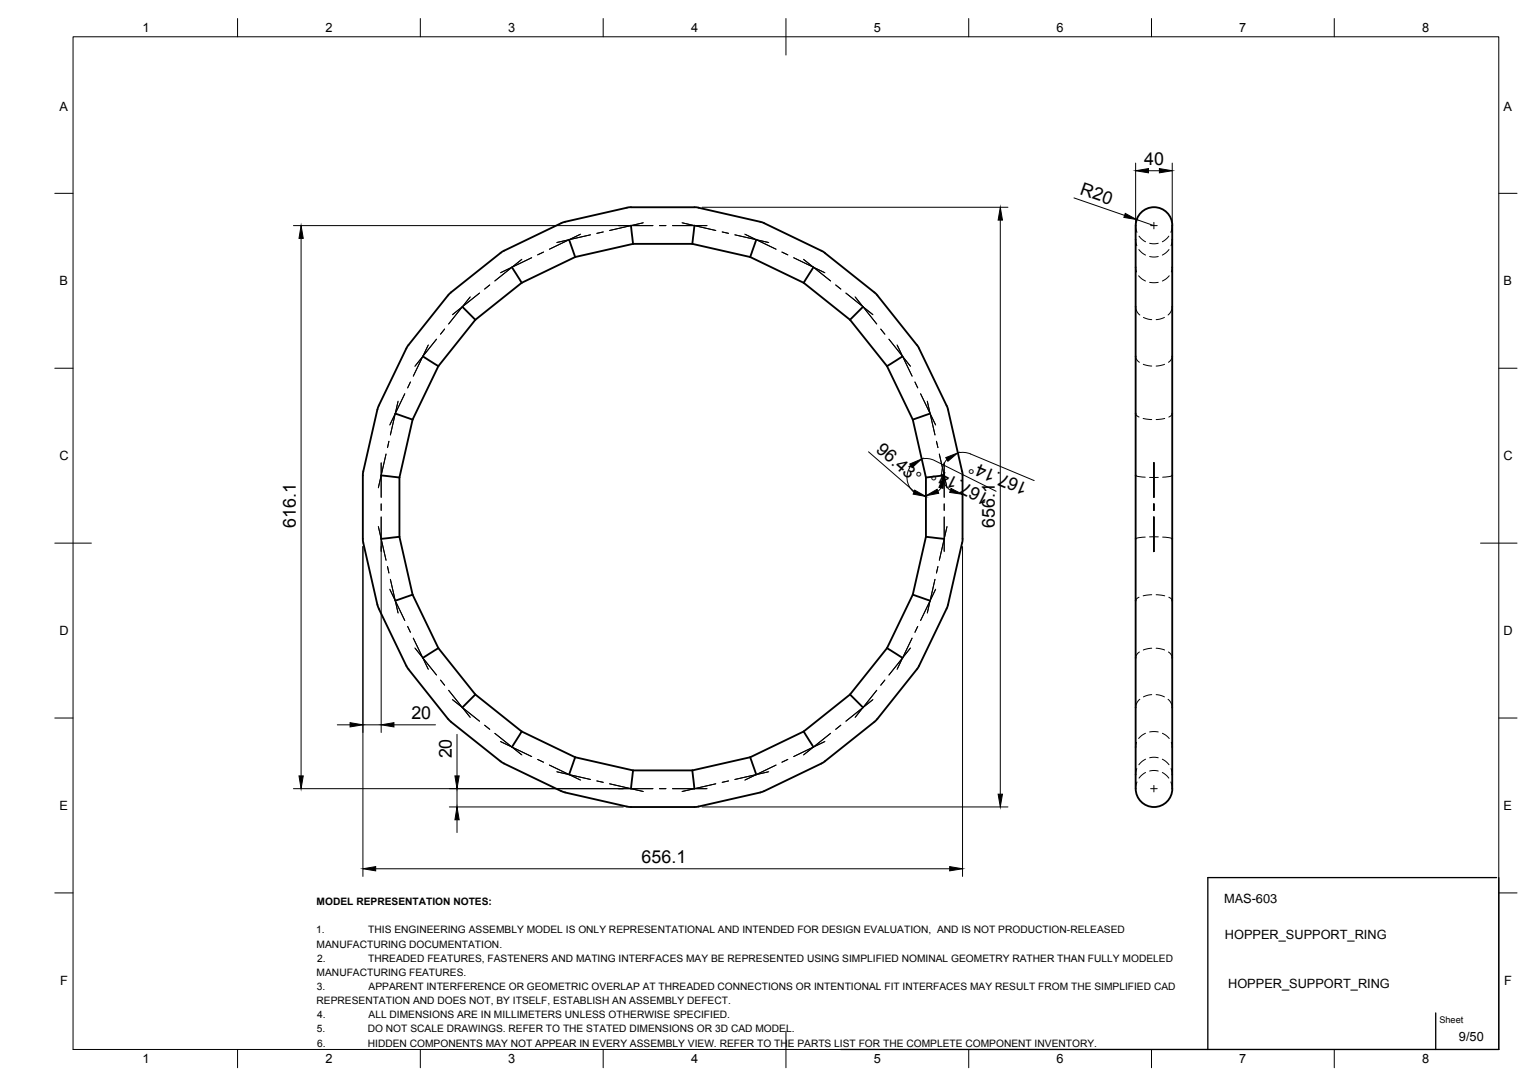
ISO-10303-21;
HEADER;
FILE_DESCRIPTION((''),'2;1');
FILE_NAME('HOPPER_SUPPORT_RING.step','2026-10-01T22:06:14-07:00',(''),(''),'','','');
FILE_SCHEMA (('AUTOMOTIVE_DESIGN { 1 0 10303 214 3 1 1 }'));
ENDSEC;
DATA;
#10=MECHANICAL_DESIGN_GEOMETRIC_PRESENTATION_REPRESENTATION('',(#985),#50440);
#362=ELLIPSE('',#29844,2.01265515316035,2.) ;
#363=ELLIPSE('',#29845,2.01265515316035,2.) ;
#364=ELLIPSE('',#29846,2.01265515316036,2.) ;
#365=ELLIPSE('',#29847,2.01265515316036,2.) ;
#366=ELLIPSE('',#29849,2.01265515316036,2.) ;
#367=ELLIPSE('',#29850,2.01265515316036,2.) ;
#368=ELLIPSE('',#29852,2.01265515316036,2.) ;
#369=ELLIPSE('',#29853,2.01265515316036,2.) ;
#370=ELLIPSE('',#29855,2.01265515316035,2.) ;
#371=ELLIPSE('',#29856,2.01265515316035,2.) ;
#372=ELLIPSE('',#29858,2.01265515316036,2.) ;
#373=ELLIPSE('',#29859,2.01265515316036,2.) ;
#374=ELLIPSE('',#29861,2.01265515316036,2.) ;
#375=ELLIPSE('',#29862,2.01265515316036,2.) ;
#376=ELLIPSE('',#29864,2.01265515316036,2.) ;
#377=ELLIPSE('',#29865,2.01265515316036,2.) ;
#378=ELLIPSE('',#29867,2.01265515316036,2.) ;
#379=ELLIPSE('',#29869,2.01265515316036,2.) ;
#380=ELLIPSE('',#29871,2.01265515316036,2.) ;
#381=ELLIPSE('',#29873,2.01265515316035,2.) ;
#382=ELLIPSE('',#29875,2.01265515316036,2.) ;
#383=ELLIPSE('',#29877,2.01265515316036,2.) ;
#384=ELLIPSE('',#29879,2.01265515316036,2.) ;
#385=ELLIPSE('',#29881,2.01265515316036,2.) ;
#386=ELLIPSE('',#29883,2.01265515316036,2.) ;
#387=ELLIPSE('',#29885,2.01265515316036,2.) ;
#388=ELLIPSE('',#29887,2.01265515316036,2.) ;
#389=ELLIPSE('',#29889,2.01265515316036,2.) ;
#390=ELLIPSE('',#29891,2.01265515316036,2.) ;
#391=ELLIPSE('',#29893,2.01265515316036,2.) ;
#392=ELLIPSE('',#29894,2.01265515316036,2.) ;
#393=ELLIPSE('',#29896,2.01265515316036,2.) ;
#394=ELLIPSE('',#29897,2.01265515316036,2.) ;
#395=ELLIPSE('',#29899,2.01265515316035,2.) ;
#396=ELLIPSE('',#29900,2.01265515316035,2.) ;
#397=ELLIPSE('',#29902,2.01265515316036,2.) ;
#398=ELLIPSE('',#29903,2.01265515316036,2.) ;
#399=ELLIPSE('',#29905,2.01265515316036,2.) ;
#400=ELLIPSE('',#29906,2.01265515316036,2.) ;
#401=ELLIPSE('',#29908,2.01265515316036,2.) ;
#402=ELLIPSE('',#29909,2.01265515316036,2.) ;
#403=ELLIPSE('',#29911,2.01265515316036,2.) ;
#404=ELLIPSE('',#29912,2.01265515316036,2.) ;
#699=SPHERICAL_SURFACE('',#29731,2.) ;
#700=SPHERICAL_SURFACE('',#29734,2.) ;
#701=SPHERICAL_SURFACE('',#29737,2.) ;
#702=SPHERICAL_SURFACE('',#29740,2.) ;
#703=SPHERICAL_SURFACE('',#29743,2.) ;
#704=SPHERICAL_SURFACE('',#29746,2.) ;
#705=SPHERICAL_SURFACE('',#29749,2.) ;
#706=SPHERICAL_SURFACE('',#29752,2.) ;
#707=SPHERICAL_SURFACE('',#29756,2.) ;
#708=SPHERICAL_SURFACE('',#29761,2.) ;
#709=SPHERICAL_SURFACE('',#29766,2.) ;
#710=SPHERICAL_SURFACE('',#29771,2.) ;
#711=SPHERICAL_SURFACE('',#29776,2.) ;
#712=SPHERICAL_SURFACE('',#29781,2.) ;
#713=SPHERICAL_SURFACE('',#29786,2.) ;
#714=SPHERICAL_SURFACE('',#29791,2.) ;
#715=SPHERICAL_SURFACE('',#29796,2.) ;
#716=SPHERICAL_SURFACE('',#29801,2.) ;
#717=SPHERICAL_SURFACE('',#29806,2.) ;
#718=SPHERICAL_SURFACE('',#29811,2.) ;
#719=SPHERICAL_SURFACE('',#29816,2.) ;
#720=SPHERICAL_SURFACE('',#29821,2.) ;
#721=SPHERICAL_SURFACE('',#29825,2.) ;
#722=SPHERICAL_SURFACE('',#29828,2.) ;
#723=SPHERICAL_SURFACE('',#29831,2.) ;
#724=SPHERICAL_SURFACE('',#29834,2.) ;
#725=SPHERICAL_SURFACE('',#29837,2.) ;
#726=SPHERICAL_SURFACE('',#29840,2.) ;
#895=SHAPE_REPRESENTATION_RELATIONSHIP('SRR','None',#50625,#940) ;
#940=ADVANCED_BREP_SHAPE_REPRESENTATION('',(#1041),#50394) ;
#985=STYLED_ITEM('',(#50883),#1041) ;
#1041=MANIFOLD_SOLID_BREP('HOPPER_SUPPORT_RING',#28633) ;
#2719=FACE_OUTER_BOUND('',#4395,.T.) ;
#2720=FACE_OUTER_BOUND('',#4396,.T.) ;
#2721=FACE_OUTER_BOUND('',#4397,.T.) ;
#2722=FACE_OUTER_BOUND('',#4398,.T.) ;
#2723=FACE_OUTER_BOUND('',#4399,.T.) ;
#2724=FACE_OUTER_BOUND('',#4400,.T.) ;
#2725=FACE_OUTER_BOUND('',#4401,.T.) ;
#2726=FACE_OUTER_BOUND('',#4402,.T.) ;
#2727=FACE_OUTER_BOUND('',#4403,.T.) ;
#2728=FACE_OUTER_BOUND('',#4404,.T.) ;
#2729=FACE_OUTER_BOUND('',#4405,.T.) ;
#2730=FACE_OUTER_BOUND('',#4406,.T.) ;
#2731=FACE_OUTER_BOUND('',#4407,.T.) ;
#2732=FACE_OUTER_BOUND('',#4408,.T.) ;
#2733=FACE_OUTER_BOUND('',#4409,.T.) ;
#2734=FACE_OUTER_BOUND('',#4410,.T.) ;
#2735=FACE_OUTER_BOUND('',#4411,.T.) ;
#2736=FACE_OUTER_BOUND('',#4412,.T.) ;
#2737=FACE_OUTER_BOUND('',#4413,.T.) ;
#2738=FACE_OUTER_BOUND('',#4414,.T.) ;
#2739=FACE_OUTER_BOUND('',#4415,.T.) ;
#2740=FACE_OUTER_BOUND('',#4416,.T.) ;
#2741=FACE_OUTER_BOUND('',#4417,.T.) ;
#2742=FACE_OUTER_BOUND('',#4418,.T.) ;
#2743=FACE_OUTER_BOUND('',#4419,.T.) ;
#2744=FACE_OUTER_BOUND('',#4420,.T.) ;
#2745=FACE_OUTER_BOUND('',#4421,.T.) ;
#2746=FACE_OUTER_BOUND('',#4422,.T.) ;
#2747=FACE_OUTER_BOUND('',#4423,.T.) ;
#2748=FACE_OUTER_BOUND('',#4424,.T.) ;
#2749=FACE_OUTER_BOUND('',#4425,.T.) ;
#2750=FACE_OUTER_BOUND('',#4426,.T.) ;
#2751=FACE_OUTER_BOUND('',#4427,.T.) ;
#2752=FACE_OUTER_BOUND('',#4428,.T.) ;
#2753=FACE_OUTER_BOUND('',#4429,.T.) ;
#2754=FACE_OUTER_BOUND('',#4430,.T.) ;
#2755=FACE_OUTER_BOUND('',#4431,.T.) ;
#2756=FACE_OUTER_BOUND('',#4432,.T.) ;
#2757=FACE_OUTER_BOUND('',#4433,.T.) ;
#2758=FACE_OUTER_BOUND('',#4434,.T.) ;
#2759=FACE_OUTER_BOUND('',#4435,.T.) ;
#2760=FACE_OUTER_BOUND('',#4436,.T.) ;
#2761=FACE_OUTER_BOUND('',#4437,.T.) ;
#2762=FACE_OUTER_BOUND('',#4438,.T.) ;
#2763=FACE_OUTER_BOUND('',#4439,.T.) ;
#2764=FACE_OUTER_BOUND('',#4440,.T.) ;
#2765=FACE_OUTER_BOUND('',#4441,.T.) ;
#2766=FACE_OUTER_BOUND('',#4442,.T.) ;
#2767=FACE_OUTER_BOUND('',#4443,.T.) ;
#2768=FACE_OUTER_BOUND('',#4444,.T.) ;
#2769=FACE_OUTER_BOUND('',#4445,.T.) ;
#2770=FACE_OUTER_BOUND('',#4446,.T.) ;
#2771=FACE_OUTER_BOUND('',#4447,.T.) ;
#2772=FACE_OUTER_BOUND('',#4448,.T.) ;
#2773=FACE_OUTER_BOUND('',#4449,.T.) ;
#2774=FACE_OUTER_BOUND('',#4450,.T.) ;
#4395=EDGE_LOOP('',(#20753,#20754)) ;
#4396=EDGE_LOOP('',(#20755,#20756)) ;
#4397=EDGE_LOOP('',(#20757,#20758)) ;
#4398=EDGE_LOOP('',(#20759,#20760)) ;
#4399=EDGE_LOOP('',(#20761,#20762)) ;
#4400=EDGE_LOOP('',(#20763,#20764)) ;
#4401=EDGE_LOOP('',(#20765,#20766)) ;
#4402=EDGE_LOOP('',(#20767,#20768,#20769)) ;
#4403=EDGE_LOOP('',(#20770,#20771,#20772,#20773)) ;
#4404=EDGE_LOOP('',(#20774,#20775,#20776,#20777)) ;
#4405=EDGE_LOOP('',(#20778,#20779,#20780,#20781)) ;
#4406=EDGE_LOOP('',(#20782,#20783,#20784,#20785)) ;
#4407=EDGE_LOOP('',(#20786,#20787,#20788,#20789)) ;
#4408=EDGE_LOOP('',(#20790,#20791,#20792,#20793)) ;
#4409=EDGE_LOOP('',(#20794,#20795,#20796,#20797)) ;
#4410=EDGE_LOOP('',(#20798,#20799,#20800,#20801)) ;
#4411=EDGE_LOOP('',(#20802,#20803,#20804,#20805)) ;
#4412=EDGE_LOOP('',(#20806,#20807,#20808,#20809)) ;
#4413=EDGE_LOOP('',(#20810,#20811,#20812,#20813)) ;
#4414=EDGE_LOOP('',(#20814,#20815,#20816,#20817)) ;
#4415=EDGE_LOOP('',(#20818,#20819,#20820,#20821)) ;
#4416=EDGE_LOOP('',(#20822,#20823,#20824)) ;
#4417=EDGE_LOOP('',(#20825,#20826)) ;
#4418=EDGE_LOOP('',(#20827,#20828)) ;
#4419=EDGE_LOOP('',(#20829,#20830)) ;
#4420=EDGE_LOOP('',(#20831,#20832)) ;
#4421=EDGE_LOOP('',(#20833,#20834)) ;
#4422=EDGE_LOOP('',(#20835,#20836)) ;
#4423=EDGE_LOOP('',(#20837,#20838,#20839,#20840,#20841,#20842,#20843,#20844)) ;
#4424=EDGE_LOOP('',(#20845,#20846,#20847,#20848,#20849,#20850,#20851,#20852)) ;
#4425=EDGE_LOOP('',(#20853,#20854,#20855,#20856,#20857,#20858,#20859,#20860)) ;
#4426=EDGE_LOOP('',(#20861,#20862,#20863,#20864,#20865,#20866,#20867,#20868)) ;
#4427=EDGE_LOOP('',(#20869,#20870,#20871,#20872,#20873,#20874,#20875,#20876)) ;
#4428=EDGE_LOOP('',(#20877,#20878,#20879,#20880,#20881,#20882,#20883,#20884)) ;
#4429=EDGE_LOOP('',(#20885,#20886,#20887,#20888,#20889,#20890,#20891,#20892)) ;
#4430=EDGE_LOOP('',(#20893,#20894,#20895,#20896,#20897,#20898,#20899,#20900,
#20901)) ;
#4431=EDGE_LOOP('',(#20902,#20903,#20904,#20905,#20906,#20907,#20908,#20909)) ;
#4432=EDGE_LOOP('',(#20910,#20911,#20912,#20913,#20914,#20915,#20916,#20917)) ;
#4433=EDGE_LOOP('',(#20918,#20919,#20920,#20921,#20922,#20923,#20924,#20925)) ;
#4434=EDGE_LOOP('',(#20926,#20927,#20928,#20929,#20930,#20931,#20932,#20933)) ;
#4435=EDGE_LOOP('',(#20934,#20935,#20936,#20937,#20938,#20939,#20940,#20941)) ;
#4436=EDGE_LOOP('',(#20942,#20943,#20944,#20945,#20946,#20947,#20948,#20949)) ;
#4437=EDGE_LOOP('',(#20950,#20951,#20952,#20953,#20954,#20955,#20956,#20957)) ;
#4438=EDGE_LOOP('',(#20958,#20959,#20960,#20961,#20962,#20963,#20964,#20965)) ;
#4439=EDGE_LOOP('',(#20966,#20967,#20968,#20969,#20970,#20971,#20972,#20973)) ;
#4440=EDGE_LOOP('',(#20974,#20975,#20976,#20977,#20978,#20979,#20980,#20981)) ;
#4441=EDGE_LOOP('',(#20982,#20983,#20984,#20985,#20986,#20987,#20988,#20989)) ;
#4442=EDGE_LOOP('',(#20990,#20991,#20992,#20993,#20994,#20995,#20996,#20997)) ;
#4443=EDGE_LOOP('',(#20998,#20999,#21000,#21001,#21002,#21003,#21004,#21005,
#21006)) ;
#4444=EDGE_LOOP('',(#21007,#21008,#21009,#21010,#21011,#21012,#21013,#21014)) ;
#4445=EDGE_LOOP('',(#21015,#21016,#21017,#21018,#21019,#21020,#21021,#21022)) ;
#4446=EDGE_LOOP('',(#21023,#21024,#21025,#21026,#21027,#21028,#21029,#21030)) ;
#4447=EDGE_LOOP('',(#21031,#21032,#21033,#21034,#21035,#21036,#21037,#21038)) ;
#4448=EDGE_LOOP('',(#21039,#21040,#21041,#21042,#21043,#21044,#21045,#21046)) ;
#4449=EDGE_LOOP('',(#21047,#21048,#21049,#21050,#21051,#21052,#21053,#21054)) ;
#4450=EDGE_LOOP('',(#21055,#21056,#21057,#21058,#21059,#21060,#21061,#21062)) ;
#6675=LINE('',#43643,#9147) ;
#6676=LINE('',#43648,#9148) ;
#6677=LINE('',#43653,#9149) ;
#6678=LINE('',#43658,#9150) ;
#6679=LINE('',#43663,#9151) ;
#6680=LINE('',#43668,#9152) ;
#6681=LINE('',#43673,#9153) ;
#6682=LINE('',#43677,#9154) ;
#6683=LINE('',#43680,#9155) ;
#6684=LINE('',#43683,#9156) ;
#6685=LINE('',#43686,#9157) ;
#6686=LINE('',#43689,#9158) ;
#6687=LINE('',#43692,#9159) ;
#6688=LINE('',#43695,#9160) ;
#6689=LINE('',#43698,#9161) ;
#6690=LINE('',#43701,#9162) ;
#6691=LINE('',#43704,#9163) ;
#6692=LINE('',#43707,#9164) ;
#6693=LINE('',#43710,#9165) ;
#6694=LINE('',#43713,#9166) ;
#6695=LINE('',#43716,#9167) ;
#6696=LINE('',#43722,#9168) ;
#6697=LINE('',#43727,#9169) ;
#6698=LINE('',#43732,#9170) ;
#6699=LINE('',#43737,#9171) ;
#6700=LINE('',#43742,#9172) ;
#6701=LINE('',#43747,#9173) ;
#6702=LINE('',#43751,#9174) ;
#9147=VECTOR('',#34592,2.) ;
#9148=VECTOR('',#34599,2.) ;
#9149=VECTOR('',#34606,2.) ;
#9150=VECTOR('',#34613,2.) ;
#9151=VECTOR('',#34620,2.) ;
#9152=VECTOR('',#34627,2.) ;
#9153=VECTOR('',#34634,2.) ;
#9154=VECTOR('',#34641,2.) ;
#9155=VECTOR('',#34646,2.) ;
#9156=VECTOR('',#34651,2.) ;
#9157=VECTOR('',#34656,2.) ;
#9158=VECTOR('',#34661,2.) ;
#9159=VECTOR('',#34666,2.) ;
#9160=VECTOR('',#34671,2.) ;
#9161=VECTOR('',#34676,2.) ;
#9162=VECTOR('',#34681,2.) ;
#9163=VECTOR('',#34686,2.) ;
#9164=VECTOR('',#34691,2.) ;
#9165=VECTOR('',#34696,2.) ;
#9166=VECTOR('',#34701,2.) ;
#9167=VECTOR('',#34706,2.) ;
#9168=VECTOR('',#34713,2.) ;
#9169=VECTOR('',#34720,2.) ;
#9170=VECTOR('',#34727,2.) ;
#9171=VECTOR('',#34734,2.) ;
#9172=VECTOR('',#34741,2.) ;
#9173=VECTOR('',#34748,2.) ;
#9174=VECTOR('',#34755,2.) ;
#10822=CIRCLE('',#29732,2.) ;
#10823=CIRCLE('',#29733,2.) ;
#10824=CIRCLE('',#29735,2.) ;
#10825=CIRCLE('',#29736,2.) ;
#10826=CIRCLE('',#29738,2.) ;
#10827=CIRCLE('',#29739,2.) ;
#10828=CIRCLE('',#29741,2.) ;
#10829=CIRCLE('',#29742,2.) ;
#10830=CIRCLE('',#29744,2.) ;
#10831=CIRCLE('',#29745,2.) ;
#10832=CIRCLE('',#29747,2.) ;
#10833=CIRCLE('',#29748,2.) ;
#10834=CIRCLE('',#29750,2.) ;
#10835=CIRCLE('',#29751,2.) ;
#10836=CIRCLE('',#29753,2.) ;
#10837=CIRCLE('',#29754,2.) ;
#10838=CIRCLE('',#29755,2.) ;
#10839=CIRCLE('',#29757,2.) ;
#10840=CIRCLE('',#29758,2.) ;
#10841=CIRCLE('',#29759,2.) ;
#10842=CIRCLE('',#29760,2.) ;
#10843=CIRCLE('',#29762,2.) ;
#10844=CIRCLE('',#29763,2.) ;
#10845=CIRCLE('',#29764,2.) ;
#10846=CIRCLE('',#29765,2.) ;
#10847=CIRCLE('',#29767,2.) ;
#10848=CIRCLE('',#29768,2.) ;
#10849=CIRCLE('',#29769,2.) ;
#10850=CIRCLE('',#29770,2.) ;
#10851=CIRCLE('',#29772,2.) ;
#10852=CIRCLE('',#29773,2.) ;
#10853=CIRCLE('',#29774,2.) ;
#10854=CIRCLE('',#29775,2.) ;
#10855=CIRCLE('',#29777,2.) ;
#10856=CIRCLE('',#29778,2.) ;
#10857=CIRCLE('',#29779,2.) ;
#10858=CIRCLE('',#29780,2.) ;
#10859=CIRCLE('',#29782,2.) ;
#10860=CIRCLE('',#29783,2.) ;
#10861=CIRCLE('',#29784,2.) ;
#10862=CIRCLE('',#29785,2.) ;
#10863=CIRCLE('',#29787,2.) ;
#10864=CIRCLE('',#29788,2.) ;
#10865=CIRCLE('',#29789,2.) ;
#10866=CIRCLE('',#29790,2.) ;
#10867=CIRCLE('',#29792,2.) ;
#10868=CIRCLE('',#29793,2.) ;
#10869=CIRCLE('',#29794,2.) ;
#10870=CIRCLE('',#29795,2.) ;
#10871=CIRCLE('',#29797,2.) ;
#10872=CIRCLE('',#29798,2.) ;
#10873=CIRCLE('',#29799,2.) ;
#10874=CIRCLE('',#29800,2.) ;
#10875=CIRCLE('',#29802,2.) ;
#10876=CIRCLE('',#29803,2.) ;
#10877=CIRCLE('',#29804,2.) ;
#10878=CIRCLE('',#29805,2.) ;
#10879=CIRCLE('',#29807,2.) ;
#10880=CIRCLE('',#29808,2.) ;
#10881=CIRCLE('',#29809,2.) ;
#10882=CIRCLE('',#29810,2.) ;
#10883=CIRCLE('',#29812,2.) ;
#10884=CIRCLE('',#29813,2.) ;
#10885=CIRCLE('',#29814,2.) ;
#10886=CIRCLE('',#29815,2.) ;
#10887=CIRCLE('',#29817,2.) ;
#10888=CIRCLE('',#29818,2.) ;
#10889=CIRCLE('',#29819,2.) ;
#10890=CIRCLE('',#29820,2.) ;
#10891=CIRCLE('',#29822,2.) ;
#10892=CIRCLE('',#29823,2.) ;
#10893=CIRCLE('',#29824,2.) ;
#10894=CIRCLE('',#29826,2.) ;
#10895=CIRCLE('',#29827,2.) ;
#10896=CIRCLE('',#29829,2.) ;
#10897=CIRCLE('',#29830,2.) ;
#10898=CIRCLE('',#29832,2.) ;
#10899=CIRCLE('',#29833,2.) ;
#10900=CIRCLE('',#29835,2.) ;
#10901=CIRCLE('',#29836,2.) ;
#10902=CIRCLE('',#29838,2.) ;
#10903=CIRCLE('',#29839,2.) ;
#10904=CIRCLE('',#29841,2.) ;
#10905=CIRCLE('',#29842,2.) ;
#12575=VERTEX_POINT('',#43443) ;
#12576=VERTEX_POINT('',#43444) ;
#12577=VERTEX_POINT('',#43448) ;
#12578=VERTEX_POINT('',#43449) ;
#12579=VERTEX_POINT('',#43453) ;
#12580=VERTEX_POINT('',#43454) ;
#12581=VERTEX_POINT('',#43458) ;
#12582=VERTEX_POINT('',#43459) ;
#12583=VERTEX_POINT('',#43463) ;
#12584=VERTEX_POINT('',#43464) ;
#12585=VERTEX_POINT('',#43468) ;
#12586=VERTEX_POINT('',#43469) ;
#12587=VERTEX_POINT('',#43473) ;
#12588=VERTEX_POINT('',#43474) ;
#12589=VERTEX_POINT('',#43478) ;
#12590=VERTEX_POINT('',#43479) ;
#12591=VERTEX_POINT('',#43481) ;
#12592=VERTEX_POINT('',#43485) ;
#12593=VERTEX_POINT('',#43486) ;
#12594=VERTEX_POINT('',#43488) ;
#12595=VERTEX_POINT('',#43490) ;
#12596=VERTEX_POINT('',#43494) ;
#12597=VERTEX_POINT('',#43495) ;
#12598=VERTEX_POINT('',#43497) ;
#12599=VERTEX_POINT('',#43499) ;
#12600=VERTEX_POINT('',#43503) ;
#12601=VERTEX_POINT('',#43504) ;
#12602=VERTEX_POINT('',#43506) ;
#12603=VERTEX_POINT('',#43508) ;
#12604=VERTEX_POINT('',#43512) ;
#12605=VERTEX_POINT('',#43513) ;
#12606=VERTEX_POINT('',#43515) ;
#12607=VERTEX_POINT('',#43517) ;
#12608=VERTEX_POINT('',#43521) ;
#12609=VERTEX_POINT('',#43522) ;
#12610=VERTEX_POINT('',#43524) ;
#12611=VERTEX_POINT('',#43526) ;
#12612=VERTEX_POINT('',#43530) ;
#12613=VERTEX_POINT('',#43531) ;
#12614=VERTEX_POINT('',#43533) ;
#12615=VERTEX_POINT('',#43535) ;
#12616=VERTEX_POINT('',#43539) ;
#12617=VERTEX_POINT('',#43540) ;
#12618=VERTEX_POINT('',#43542) ;
#12619=VERTEX_POINT('',#43544) ;
#12620=VERTEX_POINT('',#43548) ;
#12621=VERTEX_POINT('',#43549) ;
#12622=VERTEX_POINT('',#43551) ;
#12623=VERTEX_POINT('',#43553) ;
#12624=VERTEX_POINT('',#43557) ;
#12625=VERTEX_POINT('',#43558) ;
#12626=VERTEX_POINT('',#43560) ;
#12627=VERTEX_POINT('',#43562) ;
#12628=VERTEX_POINT('',#43566) ;
#12629=VERTEX_POINT('',#43567) ;
#12630=VERTEX_POINT('',#43569) ;
#12631=VERTEX_POINT('',#43571) ;
#12632=VERTEX_POINT('',#43575) ;
#12633=VERTEX_POINT('',#43576) ;
#12634=VERTEX_POINT('',#43578) ;
#12635=VERTEX_POINT('',#43580) ;
#12636=VERTEX_POINT('',#43584) ;
#12637=VERTEX_POINT('',#43585) ;
#12638=VERTEX_POINT('',#43587) ;
#12639=VERTEX_POINT('',#43589) ;
#12640=VERTEX_POINT('',#43593) ;
#12641=VERTEX_POINT('',#43594) ;
#12642=VERTEX_POINT('',#43596) ;
#12643=VERTEX_POINT('',#43598) ;
#12644=VERTEX_POINT('',#43602) ;
#12645=VERTEX_POINT('',#43603) ;
#12646=VERTEX_POINT('',#43605) ;
#12647=VERTEX_POINT('',#43609) ;
#12648=VERTEX_POINT('',#43610) ;
#12649=VERTEX_POINT('',#43614) ;
#12650=VERTEX_POINT('',#43615) ;
#12651=VERTEX_POINT('',#43619) ;
#12652=VERTEX_POINT('',#43620) ;
#12653=VERTEX_POINT('',#43624) ;
#12654=VERTEX_POINT('',#43625) ;
#12655=VERTEX_POINT('',#43629) ;
#12656=VERTEX_POINT('',#43630) ;
#12657=VERTEX_POINT('',#43634) ;
#12658=VERTEX_POINT('',#43635) ;
#12659=VERTEX_POINT('',#43639) ;
#12660=VERTEX_POINT('',#43642) ;
#12661=VERTEX_POINT('',#43647) ;
#12662=VERTEX_POINT('',#43652) ;
#12663=VERTEX_POINT('',#43657) ;
#12664=VERTEX_POINT('',#43662) ;
#12665=VERTEX_POINT('',#43667) ;
#12666=VERTEX_POINT('',#43672) ;
#12667=VERTEX_POINT('',#43717) ;
#12668=VERTEX_POINT('',#43721) ;
#12669=VERTEX_POINT('',#43726) ;
#12670=VERTEX_POINT('',#43731) ;
#12671=VERTEX_POINT('',#43736) ;
#12672=VERTEX_POINT('',#43741) ;
#12673=VERTEX_POINT('',#43746) ;
#15642=EDGE_CURVE('',#12575,#12576,#10822,.T.) ;
#15643=EDGE_CURVE('',#12576,#12575,#10823,.T.) ;
#15644=EDGE_CURVE('',#12577,#12578,#10824,.T.) ;
#15645=EDGE_CURVE('',#12578,#12577,#10825,.T.) ;
#15646=EDGE_CURVE('',#12579,#12580,#10826,.T.) ;
#15647=EDGE_CURVE('',#12580,#12579,#10827,.T.) ;
#15648=EDGE_CURVE('',#12581,#12582,#10828,.T.) ;
#15649=EDGE_CURVE('',#12582,#12581,#10829,.T.) ;
#15650=EDGE_CURVE('',#12583,#12584,#10830,.T.) ;
#15651=EDGE_CURVE('',#12584,#12583,#10831,.T.) ;
#15652=EDGE_CURVE('',#12585,#12586,#10832,.T.) ;
#15653=EDGE_CURVE('',#12586,#12585,#10833,.T.) ;
#15654=EDGE_CURVE('',#12587,#12588,#10834,.T.) ;
#15655=EDGE_CURVE('',#12588,#12587,#10835,.T.) ;
#15656=EDGE_CURVE('',#12589,#12590,#10836,.T.) ;
#15657=EDGE_CURVE('',#12590,#12591,#10837,.T.) ;
#15658=EDGE_CURVE('',#12591,#12589,#10838,.T.) ;
#15659=EDGE_CURVE('',#12592,#12593,#10839,.T.) ;
#15660=EDGE_CURVE('',#12593,#12594,#10840,.T.) ;
#15661=EDGE_CURVE('',#12594,#12595,#10841,.T.) ;
#15662=EDGE_CURVE('',#12595,#12592,#10842,.T.) ;
#15663=EDGE_CURVE('',#12596,#12597,#10843,.T.) ;
#15664=EDGE_CURVE('',#12597,#12598,#10844,.T.) ;
#15665=EDGE_CURVE('',#12598,#12599,#10845,.T.) ;
#15666=EDGE_CURVE('',#12599,#12596,#10846,.T.) ;
#15667=EDGE_CURVE('',#12600,#12601,#10847,.T.) ;
#15668=EDGE_CURVE('',#12601,#12602,#10848,.T.) ;
#15669=EDGE_CURVE('',#12602,#12603,#10849,.T.) ;
#15670=EDGE_CURVE('',#12603,#12600,#10850,.T.) ;
#15671=EDGE_CURVE('',#12604,#12605,#10851,.T.) ;
#15672=EDGE_CURVE('',#12605,#12606,#10852,.T.) ;
#15673=EDGE_CURVE('',#12606,#12607,#10853,.T.) ;
#15674=EDGE_CURVE('',#12607,#12604,#10854,.T.) ;
#15675=EDGE_CURVE('',#12608,#12609,#10855,.T.) ;
#15676=EDGE_CURVE('',#12609,#12610,#10856,.T.) ;
#15677=EDGE_CURVE('',#12610,#12611,#10857,.T.) ;
#15678=EDGE_CURVE('',#12611,#12608,#10858,.T.) ;
#15679=EDGE_CURVE('',#12612,#12613,#10859,.T.) ;
#15680=EDGE_CURVE('',#12613,#12614,#10860,.T.) ;
#15681=EDGE_CURVE('',#12614,#12615,#10861,.T.) ;
#15682=EDGE_CURVE('',#12615,#12612,#10862,.T.) ;
#15683=EDGE_CURVE('',#12616,#12617,#10863,.T.) ;
#15684=EDGE_CURVE('',#12617,#12618,#10864,.T.) ;
#15685=EDGE_CURVE('',#12618,#12619,#10865,.T.) ;
#15686=EDGE_CURVE('',#12619,#12616,#10866,.T.) ;
#15687=EDGE_CURVE('',#12620,#12621,#10867,.T.) ;
#15688=EDGE_CURVE('',#12621,#12622,#10868,.T.) ;
#15689=EDGE_CURVE('',#12622,#12623,#10869,.T.) ;
#15690=EDGE_CURVE('',#12623,#12620,#10870,.T.) ;
#15691=EDGE_CURVE('',#12624,#12625,#10871,.T.) ;
#15692=EDGE_CURVE('',#12625,#12626,#10872,.T.) ;
#15693=EDGE_CURVE('',#12626,#12627,#10873,.T.) ;
#15694=EDGE_CURVE('',#12627,#12624,#10874,.T.) ;
#15695=EDGE_CURVE('',#12628,#12629,#10875,.T.) ;
#15696=EDGE_CURVE('',#12629,#12630,#10876,.T.) ;
#15697=EDGE_CURVE('',#12630,#12631,#10877,.T.) ;
#15698=EDGE_CURVE('',#12631,#12628,#10878,.T.) ;
#15699=EDGE_CURVE('',#12632,#12633,#10879,.T.) ;
#15700=EDGE_CURVE('',#12633,#12634,#10880,.T.) ;
#15701=EDGE_CURVE('',#12634,#12635,#10881,.T.) ;
#15702=EDGE_CURVE('',#12635,#12632,#10882,.T.) ;
#15703=EDGE_CURVE('',#12636,#12637,#10883,.T.) ;
#15704=EDGE_CURVE('',#12637,#12638,#10884,.T.) ;
#15705=EDGE_CURVE('',#12638,#12639,#10885,.T.) ;
#15706=EDGE_CURVE('',#12639,#12636,#10886,.T.) ;
#15707=EDGE_CURVE('',#12640,#12641,#10887,.T.) ;
#15708=EDGE_CURVE('',#12641,#12642,#10888,.T.) ;
#15709=EDGE_CURVE('',#12642,#12643,#10889,.T.) ;
#15710=EDGE_CURVE('',#12643,#12640,#10890,.T.) ;
#15711=EDGE_CURVE('',#12644,#12645,#10891,.T.) ;
#15712=EDGE_CURVE('',#12645,#12646,#10892,.T.) ;
#15713=EDGE_CURVE('',#12646,#12644,#10893,.T.) ;
#15714=EDGE_CURVE('',#12647,#12648,#10894,.T.) ;
#15715=EDGE_CURVE('',#12648,#12647,#10895,.T.) ;
#15716=EDGE_CURVE('',#12649,#12650,#10896,.T.) ;
#15717=EDGE_CURVE('',#12650,#12649,#10897,.T.) ;
#15718=EDGE_CURVE('',#12651,#12652,#10898,.T.) ;
#15719=EDGE_CURVE('',#12652,#12651,#10899,.T.) ;
#15720=EDGE_CURVE('',#12653,#12654,#10900,.T.) ;
#15721=EDGE_CURVE('',#12654,#12653,#10901,.T.) ;
#15722=EDGE_CURVE('',#12655,#12656,#10902,.T.) ;
#15723=EDGE_CURVE('',#12656,#12655,#10903,.T.) ;
#15724=EDGE_CURVE('',#12657,#12658,#10904,.T.) ;
#15725=EDGE_CURVE('',#12658,#12657,#10905,.T.) ;
#15726=EDGE_CURVE('',#12576,#12659,#362,.T.) ;
#15727=EDGE_CURVE('',#12659,#12575,#363,.T.) ;
#15728=EDGE_CURVE('',#12659,#12660,#6675,.T.) ;
#15729=EDGE_CURVE('',#12578,#12660,#364,.T.) ;
#15730=EDGE_CURVE('',#12660,#12577,#365,.T.) ;
#15731=EDGE_CURVE('',#12660,#12661,#6676,.T.) ;
#15732=EDGE_CURVE('',#12580,#12661,#366,.T.) ;
#15733=EDGE_CURVE('',#12661,#12579,#367,.T.) ;
#15734=EDGE_CURVE('',#12661,#12662,#6677,.T.) ;
#15735=EDGE_CURVE('',#12582,#12662,#368,.T.) ;
#15736=EDGE_CURVE('',#12662,#12581,#369,.T.) ;
#15737=EDGE_CURVE('',#12662,#12663,#6678,.T.) ;
#15738=EDGE_CURVE('',#12584,#12663,#370,.T.) ;
#15739=EDGE_CURVE('',#12663,#12583,#371,.T.) ;
#15740=EDGE_CURVE('',#12663,#12664,#6679,.T.) ;
#15741=EDGE_CURVE('',#12586,#12664,#372,.T.) ;
#15742=EDGE_CURVE('',#12664,#12585,#373,.T.) ;
#15743=EDGE_CURVE('',#12664,#12665,#6680,.T.) ;
#15744=EDGE_CURVE('',#12588,#12665,#374,.T.) ;
#15745=EDGE_CURVE('',#12665,#12587,#375,.T.) ;
#15746=EDGE_CURVE('',#12665,#12666,#6681,.T.) ;
#15747=EDGE_CURVE('',#12590,#12666,#376,.T.) ;
#15748=EDGE_CURVE('',#12666,#12589,#377,.T.) ;
#15749=EDGE_CURVE('',#12591,#12593,#6682,.T.) ;
#15750=EDGE_CURVE('',#12594,#12592,#378,.T.) ;
#15751=EDGE_CURVE('',#12595,#12597,#6683,.T.) ;
#15752=EDGE_CURVE('',#12598,#12596,#379,.T.) ;
#15753=EDGE_CURVE('',#12599,#12601,#6684,.T.) ;
#15754=EDGE_CURVE('',#12602,#12600,#380,.T.) ;
#15755=EDGE_CURVE('',#12603,#12605,#6685,.T.) ;
#15756=EDGE_CURVE('',#12606,#12604,#381,.T.) ;
#15757=EDGE_CURVE('',#12607,#12609,#6686,.T.) ;
#15758=EDGE_CURVE('',#12610,#12608,#382,.T.) ;
#15759=EDGE_CURVE('',#12611,#12613,#6687,.T.) ;
#15760=EDGE_CURVE('',#12614,#12612,#383,.T.) ;
#15761=EDGE_CURVE('',#12615,#12617,#6688,.T.) ;
#15762=EDGE_CURVE('',#12618,#12616,#384,.T.) ;
#15763=EDGE_CURVE('',#12619,#12621,#6689,.T.) ;
#15764=EDGE_CURVE('',#12622,#12620,#385,.T.) ;
#15765=EDGE_CURVE('',#12623,#12625,#6690,.T.) ;
#15766=EDGE_CURVE('',#12626,#12624,#386,.T.) ;
#15767=EDGE_CURVE('',#12627,#12629,#6691,.T.) ;
#15768=EDGE_CURVE('',#12630,#12628,#387,.T.) ;
#15769=EDGE_CURVE('',#12631,#12633,#6692,.T.) ;
#15770=EDGE_CURVE('',#12634,#12632,#388,.T.) ;
#15771=EDGE_CURVE('',#12635,#12637,#6693,.T.) ;
#15772=EDGE_CURVE('',#12638,#12636,#389,.T.) ;
#15773=EDGE_CURVE('',#12639,#12641,#6694,.T.) ;
#15774=EDGE_CURVE('',#12642,#12640,#390,.T.) ;
#15775=EDGE_CURVE('',#12643,#12645,#6695,.T.) ;
#15776=EDGE_CURVE('',#12667,#12644,#391,.T.) ;
#15777=EDGE_CURVE('',#12646,#12667,#392,.T.) ;
#15778=EDGE_CURVE('',#12667,#12668,#6696,.T.) ;
#15779=EDGE_CURVE('',#12648,#12668,#393,.T.) ;
#15780=EDGE_CURVE('',#12668,#12647,#394,.T.) ;
#15781=EDGE_CURVE('',#12668,#12669,#6697,.T.) ;
#15782=EDGE_CURVE('',#12650,#12669,#395,.T.) ;
#15783=EDGE_CURVE('',#12669,#12649,#396,.T.) ;
#15784=EDGE_CURVE('',#12669,#12670,#6698,.T.) ;
#15785=EDGE_CURVE('',#12652,#12670,#397,.T.) ;
#15786=EDGE_CURVE('',#12670,#12651,#398,.T.) ;
#15787=EDGE_CURVE('',#12670,#12671,#6699,.T.) ;
#15788=EDGE_CURVE('',#12654,#12671,#399,.T.) ;
#15789=EDGE_CURVE('',#12671,#12653,#400,.T.) ;
#15790=EDGE_CURVE('',#12671,#12672,#6700,.T.) ;
#15791=EDGE_CURVE('',#12656,#12672,#401,.T.) ;
#15792=EDGE_CURVE('',#12672,#12655,#402,.T.) ;
#15793=EDGE_CURVE('',#12672,#12673,#6701,.T.) ;
#15794=EDGE_CURVE('',#12658,#12673,#403,.T.) ;
#15795=EDGE_CURVE('',#12673,#12657,#404,.T.) ;
#15796=EDGE_CURVE('',#12673,#12659,#6702,.T.) ;
#20753=ORIENTED_EDGE('',*,*,#15642,.T.) ;
#20754=ORIENTED_EDGE('',*,*,#15643,.T.) ;
#20755=ORIENTED_EDGE('',*,*,#15644,.T.) ;
#20756=ORIENTED_EDGE('',*,*,#15645,.T.) ;
#20757=ORIENTED_EDGE('',*,*,#15646,.T.) ;
#20758=ORIENTED_EDGE('',*,*,#15647,.T.) ;
#20759=ORIENTED_EDGE('',*,*,#15648,.T.) ;
#20760=ORIENTED_EDGE('',*,*,#15649,.T.) ;
#20761=ORIENTED_EDGE('',*,*,#15650,.T.) ;
#20762=ORIENTED_EDGE('',*,*,#15651,.T.) ;
#20763=ORIENTED_EDGE('',*,*,#15652,.T.) ;
#20764=ORIENTED_EDGE('',*,*,#15653,.T.) ;
#20765=ORIENTED_EDGE('',*,*,#15654,.T.) ;
#20766=ORIENTED_EDGE('',*,*,#15655,.T.) ;
#20767=ORIENTED_EDGE('',*,*,#15656,.T.) ;
#20768=ORIENTED_EDGE('',*,*,#15657,.T.) ;
#20769=ORIENTED_EDGE('',*,*,#15658,.T.) ;
#20770=ORIENTED_EDGE('',*,*,#15659,.T.) ;
#20771=ORIENTED_EDGE('',*,*,#15660,.T.) ;
#20772=ORIENTED_EDGE('',*,*,#15661,.T.) ;
#20773=ORIENTED_EDGE('',*,*,#15662,.T.) ;
#20774=ORIENTED_EDGE('',*,*,#15663,.T.) ;
#20775=ORIENTED_EDGE('',*,*,#15664,.T.) ;
#20776=ORIENTED_EDGE('',*,*,#15665,.T.) ;
#20777=ORIENTED_EDGE('',*,*,#15666,.T.) ;
#20778=ORIENTED_EDGE('',*,*,#15667,.T.) ;
#20779=ORIENTED_EDGE('',*,*,#15668,.T.) ;
#20780=ORIENTED_EDGE('',*,*,#15669,.T.) ;
#20781=ORIENTED_EDGE('',*,*,#15670,.T.) ;
#20782=ORIENTED_EDGE('',*,*,#15671,.T.) ;
#20783=ORIENTED_EDGE('',*,*,#15672,.T.) ;
#20784=ORIENTED_EDGE('',*,*,#15673,.T.) ;
#20785=ORIENTED_EDGE('',*,*,#15674,.T.) ;
#20786=ORIENTED_EDGE('',*,*,#15675,.T.) ;
#20787=ORIENTED_EDGE('',*,*,#15676,.T.) ;
#20788=ORIENTED_EDGE('',*,*,#15677,.T.) ;
#20789=ORIENTED_EDGE('',*,*,#15678,.T.) ;
#20790=ORIENTED_EDGE('',*,*,#15679,.T.) ;
#20791=ORIENTED_EDGE('',*,*,#15680,.T.) ;
#20792=ORIENTED_EDGE('',*,*,#15681,.T.) ;
#20793=ORIENTED_EDGE('',*,*,#15682,.T.) ;
#20794=ORIENTED_EDGE('',*,*,#15683,.T.) ;
#20795=ORIENTED_EDGE('',*,*,#15684,.T.) ;
#20796=ORIENTED_EDGE('',*,*,#15685,.T.) ;
#20797=ORIENTED_EDGE('',*,*,#15686,.T.) ;
#20798=ORIENTED_EDGE('',*,*,#15687,.T.) ;
#20799=ORIENTED_EDGE('',*,*,#15688,.T.) ;
#20800=ORIENTED_EDGE('',*,*,#15689,.T.) ;
#20801=ORIENTED_EDGE('',*,*,#15690,.T.) ;
#20802=ORIENTED_EDGE('',*,*,#15691,.T.) ;
#20803=ORIENTED_EDGE('',*,*,#15692,.T.) ;
#20804=ORIENTED_EDGE('',*,*,#15693,.T.) ;
#20805=ORIENTED_EDGE('',*,*,#15694,.T.) ;
#20806=ORIENTED_EDGE('',*,*,#15695,.T.) ;
#20807=ORIENTED_EDGE('',*,*,#15696,.T.) ;
#20808=ORIENTED_EDGE('',*,*,#15697,.T.) ;
#20809=ORIENTED_EDGE('',*,*,#15698,.T.) ;
#20810=ORIENTED_EDGE('',*,*,#15699,.T.) ;
#20811=ORIENTED_EDGE('',*,*,#15700,.T.) ;
#20812=ORIENTED_EDGE('',*,*,#15701,.T.) ;
#20813=ORIENTED_EDGE('',*,*,#15702,.T.) ;
#20814=ORIENTED_EDGE('',*,*,#15703,.T.) ;
#20815=ORIENTED_EDGE('',*,*,#15704,.T.) ;
#20816=ORIENTED_EDGE('',*,*,#15705,.T.) ;
#20817=ORIENTED_EDGE('',*,*,#15706,.T.) ;
#20818=ORIENTED_EDGE('',*,*,#15707,.T.) ;
#20819=ORIENTED_EDGE('',*,*,#15708,.T.) ;
#20820=ORIENTED_EDGE('',*,*,#15709,.T.) ;
#20821=ORIENTED_EDGE('',*,*,#15710,.T.) ;
#20822=ORIENTED_EDGE('',*,*,#15711,.T.) ;
#20823=ORIENTED_EDGE('',*,*,#15712,.T.) ;
#20824=ORIENTED_EDGE('',*,*,#15713,.T.) ;
#20825=ORIENTED_EDGE('',*,*,#15714,.T.) ;
#20826=ORIENTED_EDGE('',*,*,#15715,.T.) ;
#20827=ORIENTED_EDGE('',*,*,#15716,.T.) ;
#20828=ORIENTED_EDGE('',*,*,#15717,.T.) ;
#20829=ORIENTED_EDGE('',*,*,#15718,.T.) ;
#20830=ORIENTED_EDGE('',*,*,#15719,.T.) ;
#20831=ORIENTED_EDGE('',*,*,#15720,.T.) ;
#20832=ORIENTED_EDGE('',*,*,#15721,.T.) ;
#20833=ORIENTED_EDGE('',*,*,#15722,.T.) ;
#20834=ORIENTED_EDGE('',*,*,#15723,.T.) ;
#20835=ORIENTED_EDGE('',*,*,#15724,.T.) ;
#20836=ORIENTED_EDGE('',*,*,#15725,.T.) ;
#20837=ORIENTED_EDGE('',*,*,#15726,.F.) ;
#20838=ORIENTED_EDGE('',*,*,#15642,.F.) ;
#20839=ORIENTED_EDGE('',*,*,#15727,.F.) ;
#20840=ORIENTED_EDGE('',*,*,#15728,.T.) ;
#20841=ORIENTED_EDGE('',*,*,#15729,.F.) ;
#20842=ORIENTED_EDGE('',*,*,#15644,.F.) ;
#20843=ORIENTED_EDGE('',*,*,#15730,.F.) ;
#20844=ORIENTED_EDGE('',*,*,#15728,.F.) ;
#20845=ORIENTED_EDGE('',*,*,#15729,.T.) ;
#20846=ORIENTED_EDGE('',*,*,#15731,.T.) ;
#20847=ORIENTED_EDGE('',*,*,#15732,.F.) ;
#20848=ORIENTED_EDGE('',*,*,#15646,.F.) ;
#20849=ORIENTED_EDGE('',*,*,#15733,.F.) ;
#20850=ORIENTED_EDGE('',*,*,#15731,.F.) ;
#20851=ORIENTED_EDGE('',*,*,#15730,.T.) ;
#20852=ORIENTED_EDGE('',*,*,#15645,.F.) ;
#20853=ORIENTED_EDGE('',*,*,#15732,.T.) ;
#20854=ORIENTED_EDGE('',*,*,#15734,.T.) ;
#20855=ORIENTED_EDGE('',*,*,#15735,.F.) ;
#20856=ORIENTED_EDGE('',*,*,#15648,.F.) ;
#20857=ORIENTED_EDGE('',*,*,#15736,.F.) ;
#20858=ORIENTED_EDGE('',*,*,#15734,.F.) ;
#20859=ORIENTED_EDGE('',*,*,#15733,.T.) ;
#20860=ORIENTED_EDGE('',*,*,#15647,.F.) ;
#20861=ORIENTED_EDGE('',*,*,#15735,.T.) ;
#20862=ORIENTED_EDGE('',*,*,#15737,.T.) ;
#20863=ORIENTED_EDGE('',*,*,#15738,.F.) ;
#20864=ORIENTED_EDGE('',*,*,#15650,.F.) ;
#20865=ORIENTED_EDGE('',*,*,#15739,.F.) ;
#20866=ORIENTED_EDGE('',*,*,#15737,.F.) ;
#20867=ORIENTED_EDGE('',*,*,#15736,.T.) ;
#20868=ORIENTED_EDGE('',*,*,#15649,.F.) ;
#20869=ORIENTED_EDGE('',*,*,#15738,.T.) ;
#20870=ORIENTED_EDGE('',*,*,#15740,.T.) ;
#20871=ORIENTED_EDGE('',*,*,#15741,.F.) ;
#20872=ORIENTED_EDGE('',*,*,#15652,.F.) ;
#20873=ORIENTED_EDGE('',*,*,#15742,.F.) ;
#20874=ORIENTED_EDGE('',*,*,#15740,.F.) ;
#20875=ORIENTED_EDGE('',*,*,#15739,.T.) ;
#20876=ORIENTED_EDGE('',*,*,#15651,.F.) ;
#20877=ORIENTED_EDGE('',*,*,#15741,.T.) ;
#20878=ORIENTED_EDGE('',*,*,#15743,.T.) ;
#20879=ORIENTED_EDGE('',*,*,#15744,.F.) ;
#20880=ORIENTED_EDGE('',*,*,#15654,.F.) ;
#20881=ORIENTED_EDGE('',*,*,#15745,.F.) ;
#20882=ORIENTED_EDGE('',*,*,#15743,.F.) ;
#20883=ORIENTED_EDGE('',*,*,#15742,.T.) ;
#20884=ORIENTED_EDGE('',*,*,#15653,.F.) ;
#20885=ORIENTED_EDGE('',*,*,#15744,.T.) ;
#20886=ORIENTED_EDGE('',*,*,#15746,.T.) ;
#20887=ORIENTED_EDGE('',*,*,#15747,.F.) ;
#20888=ORIENTED_EDGE('',*,*,#15656,.F.) ;
#20889=ORIENTED_EDGE('',*,*,#15748,.F.) ;
#20890=ORIENTED_EDGE('',*,*,#15746,.F.) ;
#20891=ORIENTED_EDGE('',*,*,#15745,.T.) ;
#20892=ORIENTED_EDGE('',*,*,#15655,.F.) ;
#20893=ORIENTED_EDGE('',*,*,#15747,.T.) ;
#20894=ORIENTED_EDGE('',*,*,#15748,.T.) ;
#20895=ORIENTED_EDGE('',*,*,#15658,.F.) ;
#20896=ORIENTED_EDGE('',*,*,#15749,.T.) ;
#20897=ORIENTED_EDGE('',*,*,#15659,.F.) ;
#20898=ORIENTED_EDGE('',*,*,#15750,.F.) ;
#20899=ORIENTED_EDGE('',*,*,#15660,.F.) ;
#20900=ORIENTED_EDGE('',*,*,#15749,.F.) ;
#20901=ORIENTED_EDGE('',*,*,#15657,.F.) ;
#20902=ORIENTED_EDGE('',*,*,#15750,.T.) ;
#20903=ORIENTED_EDGE('',*,*,#15662,.F.) ;
#20904=ORIENTED_EDGE('',*,*,#15751,.T.) ;
#20905=ORIENTED_EDGE('',*,*,#15663,.F.) ;
#20906=ORIENTED_EDGE('',*,*,#15752,.F.) ;
#20907=ORIENTED_EDGE('',*,*,#15664,.F.) ;
#20908=ORIENTED_EDGE('',*,*,#15751,.F.) ;
#20909=ORIENTED_EDGE('',*,*,#15661,.F.) ;
#20910=ORIENTED_EDGE('',*,*,#15752,.T.) ;
#20911=ORIENTED_EDGE('',*,*,#15666,.F.) ;
#20912=ORIENTED_EDGE('',*,*,#15753,.T.) ;
#20913=ORIENTED_EDGE('',*,*,#15667,.F.) ;
#20914=ORIENTED_EDGE('',*,*,#15754,.F.) ;
#20915=ORIENTED_EDGE('',*,*,#15668,.F.) ;
#20916=ORIENTED_EDGE('',*,*,#15753,.F.) ;
#20917=ORIENTED_EDGE('',*,*,#15665,.F.) ;
#20918=ORIENTED_EDGE('',*,*,#15754,.T.) ;
#20919=ORIENTED_EDGE('',*,*,#15670,.F.) ;
#20920=ORIENTED_EDGE('',*,*,#15755,.T.) ;
#20921=ORIENTED_EDGE('',*,*,#15671,.F.) ;
#20922=ORIENTED_EDGE('',*,*,#15756,.F.) ;
#20923=ORIENTED_EDGE('',*,*,#15672,.F.) ;
#20924=ORIENTED_EDGE('',*,*,#15755,.F.) ;
#20925=ORIENTED_EDGE('',*,*,#15669,.F.) ;
#20926=ORIENTED_EDGE('',*,*,#15756,.T.) ;
#20927=ORIENTED_EDGE('',*,*,#15674,.F.) ;
#20928=ORIENTED_EDGE('',*,*,#15757,.T.) ;
#20929=ORIENTED_EDGE('',*,*,#15675,.F.) ;
#20930=ORIENTED_EDGE('',*,*,#15758,.F.) ;
#20931=ORIENTED_EDGE('',*,*,#15676,.F.) ;
#20932=ORIENTED_EDGE('',*,*,#15757,.F.) ;
#20933=ORIENTED_EDGE('',*,*,#15673,.F.) ;
#20934=ORIENTED_EDGE('',*,*,#15758,.T.) ;
#20935=ORIENTED_EDGE('',*,*,#15678,.F.) ;
#20936=ORIENTED_EDGE('',*,*,#15759,.T.) ;
#20937=ORIENTED_EDGE('',*,*,#15679,.F.) ;
#20938=ORIENTED_EDGE('',*,*,#15760,.F.) ;
#20939=ORIENTED_EDGE('',*,*,#15680,.F.) ;
#20940=ORIENTED_EDGE('',*,*,#15759,.F.) ;
#20941=ORIENTED_EDGE('',*,*,#15677,.F.) ;
#20942=ORIENTED_EDGE('',*,*,#15760,.T.) ;
#20943=ORIENTED_EDGE('',*,*,#15682,.F.) ;
#20944=ORIENTED_EDGE('',*,*,#15761,.T.) ;
#20945=ORIENTED_EDGE('',*,*,#15683,.F.) ;
#20946=ORIENTED_EDGE('',*,*,#15762,.F.) ;
#20947=ORIENTED_EDGE('',*,*,#15684,.F.) ;
#20948=ORIENTED_EDGE('',*,*,#15761,.F.) ;
#20949=ORIENTED_EDGE('',*,*,#15681,.F.) ;
#20950=ORIENTED_EDGE('',*,*,#15762,.T.) ;
#20951=ORIENTED_EDGE('',*,*,#15686,.F.) ;
#20952=ORIENTED_EDGE('',*,*,#15763,.T.) ;
#20953=ORIENTED_EDGE('',*,*,#15687,.F.) ;
#20954=ORIENTED_EDGE('',*,*,#15764,.F.) ;
#20955=ORIENTED_EDGE('',*,*,#15688,.F.) ;
#20956=ORIENTED_EDGE('',*,*,#15763,.F.) ;
#20957=ORIENTED_EDGE('',*,*,#15685,.F.) ;
#20958=ORIENTED_EDGE('',*,*,#15764,.T.) ;
#20959=ORIENTED_EDGE('',*,*,#15690,.F.) ;
#20960=ORIENTED_EDGE('',*,*,#15765,.T.) ;
#20961=ORIENTED_EDGE('',*,*,#15691,.F.) ;
#20962=ORIENTED_EDGE('',*,*,#15766,.F.) ;
#20963=ORIENTED_EDGE('',*,*,#15692,.F.) ;
#20964=ORIENTED_EDGE('',*,*,#15765,.F.) ;
#20965=ORIENTED_EDGE('',*,*,#15689,.F.) ;
#20966=ORIENTED_EDGE('',*,*,#15766,.T.) ;
#20967=ORIENTED_EDGE('',*,*,#15694,.F.) ;
#20968=ORIENTED_EDGE('',*,*,#15767,.T.) ;
#20969=ORIENTED_EDGE('',*,*,#15695,.F.) ;
#20970=ORIENTED_EDGE('',*,*,#15768,.F.) ;
#20971=ORIENTED_EDGE('',*,*,#15696,.F.) ;
#20972=ORIENTED_EDGE('',*,*,#15767,.F.) ;
#20973=ORIENTED_EDGE('',*,*,#15693,.F.) ;
#20974=ORIENTED_EDGE('',*,*,#15768,.T.) ;
#20975=ORIENTED_EDGE('',*,*,#15698,.F.) ;
#20976=ORIENTED_EDGE('',*,*,#15769,.T.) ;
#20977=ORIENTED_EDGE('',*,*,#15699,.F.) ;
#20978=ORIENTED_EDGE('',*,*,#15770,.F.) ;
#20979=ORIENTED_EDGE('',*,*,#15700,.F.) ;
#20980=ORIENTED_EDGE('',*,*,#15769,.F.) ;
#20981=ORIENTED_EDGE('',*,*,#15697,.F.) ;
#20982=ORIENTED_EDGE('',*,*,#15770,.T.) ;
#20983=ORIENTED_EDGE('',*,*,#15702,.F.) ;
#20984=ORIENTED_EDGE('',*,*,#15771,.T.) ;
#20985=ORIENTED_EDGE('',*,*,#15703,.F.) ;
#20986=ORIENTED_EDGE('',*,*,#15772,.F.) ;
#20987=ORIENTED_EDGE('',*,*,#15704,.F.) ;
#20988=ORIENTED_EDGE('',*,*,#15771,.F.) ;
#20989=ORIENTED_EDGE('',*,*,#15701,.F.) ;
#20990=ORIENTED_EDGE('',*,*,#15772,.T.) ;
#20991=ORIENTED_EDGE('',*,*,#15706,.F.) ;
#20992=ORIENTED_EDGE('',*,*,#15773,.T.) ;
#20993=ORIENTED_EDGE('',*,*,#15707,.F.) ;
#20994=ORIENTED_EDGE('',*,*,#15774,.F.) ;
#20995=ORIENTED_EDGE('',*,*,#15708,.F.) ;
#20996=ORIENTED_EDGE('',*,*,#15773,.F.) ;
#20997=ORIENTED_EDGE('',*,*,#15705,.F.) ;
#20998=ORIENTED_EDGE('',*,*,#15774,.T.) ;
#20999=ORIENTED_EDGE('',*,*,#15710,.F.) ;
#21000=ORIENTED_EDGE('',*,*,#15775,.T.) ;
#21001=ORIENTED_EDGE('',*,*,#15711,.F.) ;
#21002=ORIENTED_EDGE('',*,*,#15776,.F.) ;
#21003=ORIENTED_EDGE('',*,*,#15777,.F.) ;
#21004=ORIENTED_EDGE('',*,*,#15712,.F.) ;
#21005=ORIENTED_EDGE('',*,*,#15775,.F.) ;
#21006=ORIENTED_EDGE('',*,*,#15709,.F.) ;
#21007=ORIENTED_EDGE('',*,*,#15777,.T.) ;
#21008=ORIENTED_EDGE('',*,*,#15778,.T.) ;
#21009=ORIENTED_EDGE('',*,*,#15779,.F.) ;
#21010=ORIENTED_EDGE('',*,*,#15714,.F.) ;
#21011=ORIENTED_EDGE('',*,*,#15780,.F.) ;
#21012=ORIENTED_EDGE('',*,*,#15778,.F.) ;
#21013=ORIENTED_EDGE('',*,*,#15776,.T.) ;
#21014=ORIENTED_EDGE('',*,*,#15713,.F.) ;
#21015=ORIENTED_EDGE('',*,*,#15779,.T.) ;
#21016=ORIENTED_EDGE('',*,*,#15781,.T.) ;
#21017=ORIENTED_EDGE('',*,*,#15782,.F.) ;
#21018=ORIENTED_EDGE('',*,*,#15716,.F.) ;
#21019=ORIENTED_EDGE('',*,*,#15783,.F.) ;
#21020=ORIENTED_EDGE('',*,*,#15781,.F.) ;
#21021=ORIENTED_EDGE('',*,*,#15780,.T.) ;
#21022=ORIENTED_EDGE('',*,*,#15715,.F.) ;
#21023=ORIENTED_EDGE('',*,*,#15782,.T.) ;
#21024=ORIENTED_EDGE('',*,*,#15784,.T.) ;
#21025=ORIENTED_EDGE('',*,*,#15785,.F.) ;
#21026=ORIENTED_EDGE('',*,*,#15718,.F.) ;
#21027=ORIENTED_EDGE('',*,*,#15786,.F.) ;
#21028=ORIENTED_EDGE('',*,*,#15784,.F.) ;
#21029=ORIENTED_EDGE('',*,*,#15783,.T.) ;
#21030=ORIENTED_EDGE('',*,*,#15717,.F.) ;
#21031=ORIENTED_EDGE('',*,*,#15785,.T.) ;
#21032=ORIENTED_EDGE('',*,*,#15787,.T.) ;
#21033=ORIENTED_EDGE('',*,*,#15788,.F.) ;
#21034=ORIENTED_EDGE('',*,*,#15720,.F.) ;
#21035=ORIENTED_EDGE('',*,*,#15789,.F.) ;
#21036=ORIENTED_EDGE('',*,*,#15787,.F.) ;
#21037=ORIENTED_EDGE('',*,*,#15786,.T.) ;
#21038=ORIENTED_EDGE('',*,*,#15719,.F.) ;
#21039=ORIENTED_EDGE('',*,*,#15788,.T.) ;
#21040=ORIENTED_EDGE('',*,*,#15790,.T.) ;
#21041=ORIENTED_EDGE('',*,*,#15791,.F.) ;
#21042=ORIENTED_EDGE('',*,*,#15722,.F.) ;
#21043=ORIENTED_EDGE('',*,*,#15792,.F.) ;
#21044=ORIENTED_EDGE('',*,*,#15790,.F.) ;
#21045=ORIENTED_EDGE('',*,*,#15789,.T.) ;
#21046=ORIENTED_EDGE('',*,*,#15721,.F.) ;
#21047=ORIENTED_EDGE('',*,*,#15791,.T.) ;
#21048=ORIENTED_EDGE('',*,*,#15793,.T.) ;
#21049=ORIENTED_EDGE('',*,*,#15794,.F.) ;
#21050=ORIENTED_EDGE('',*,*,#15724,.F.) ;
#21051=ORIENTED_EDGE('',*,*,#15795,.F.) ;
#21052=ORIENTED_EDGE('',*,*,#15793,.F.) ;
#21053=ORIENTED_EDGE('',*,*,#15792,.T.) ;
#21054=ORIENTED_EDGE('',*,*,#15723,.F.) ;
#21055=ORIENTED_EDGE('',*,*,#15794,.T.) ;
#21056=ORIENTED_EDGE('',*,*,#15796,.T.) ;
#21057=ORIENTED_EDGE('',*,*,#15727,.T.) ;
#21058=ORIENTED_EDGE('',*,*,#15643,.F.) ;
#21059=ORIENTED_EDGE('',*,*,#15726,.T.) ;
#21060=ORIENTED_EDGE('',*,*,#15796,.F.) ;
#21061=ORIENTED_EDGE('',*,*,#15795,.T.) ;
#21062=ORIENTED_EDGE('',*,*,#15725,.F.) ;
#26707=CYLINDRICAL_SURFACE('',#29843,2.) ;
#26708=CYLINDRICAL_SURFACE('',#29848,2.) ;
#26709=CYLINDRICAL_SURFACE('',#29851,2.) ;
#26710=CYLINDRICAL_SURFACE('',#29854,2.) ;
#26711=CYLINDRICAL_SURFACE('',#29857,2.) ;
#26712=CYLINDRICAL_SURFACE('',#29860,2.) ;
#26713=CYLINDRICAL_SURFACE('',#29863,2.) ;
#26714=CYLINDRICAL_SURFACE('',#29866,2.) ;
#26715=CYLINDRICAL_SURFACE('',#29868,2.) ;
#26716=CYLINDRICAL_SURFACE('',#29870,2.) ;
#26717=CYLINDRICAL_SURFACE('',#29872,2.) ;
#26718=CYLINDRICAL_SURFACE('',#29874,2.) ;
#26719=CYLINDRICAL_SURFACE('',#29876,2.) ;
#26720=CYLINDRICAL_SURFACE('',#29878,2.) ;
#26721=CYLINDRICAL_SURFACE('',#29880,2.) ;
#26722=CYLINDRICAL_SURFACE('',#29882,2.) ;
#26723=CYLINDRICAL_SURFACE('',#29884,2.) ;
#26724=CYLINDRICAL_SURFACE('',#29886,2.) ;
#26725=CYLINDRICAL_SURFACE('',#29888,2.) ;
#26726=CYLINDRICAL_SURFACE('',#29890,2.) ;
#26727=CYLINDRICAL_SURFACE('',#29892,2.) ;
#26728=CYLINDRICAL_SURFACE('',#29895,2.) ;
#26729=CYLINDRICAL_SURFACE('',#29898,2.) ;
#26730=CYLINDRICAL_SURFACE('',#29901,2.) ;
#26731=CYLINDRICAL_SURFACE('',#29904,2.) ;
#26732=CYLINDRICAL_SURFACE('',#29907,2.) ;
#26733=CYLINDRICAL_SURFACE('',#29910,2.) ;
#26734=CYLINDRICAL_SURFACE('',#29913,2.) ;
#27454=ADVANCED_FACE('',(#2719),#699,.T.) ;
#27455=ADVANCED_FACE('',(#2720),#700,.T.) ;
#27456=ADVANCED_FACE('',(#2721),#701,.T.) ;
#27457=ADVANCED_FACE('',(#2722),#702,.T.) ;
#27458=ADVANCED_FACE('',(#2723),#703,.T.) ;
#27459=ADVANCED_FACE('',(#2724),#704,.T.) ;
#27460=ADVANCED_FACE('',(#2725),#705,.T.) ;
#27461=ADVANCED_FACE('',(#2726),#706,.T.) ;
#27462=ADVANCED_FACE('',(#2727),#707,.T.) ;
#27463=ADVANCED_FACE('',(#2728),#708,.T.) ;
#27464=ADVANCED_FACE('',(#2729),#709,.T.) ;
#27465=ADVANCED_FACE('',(#2730),#710,.T.) ;
#27466=ADVANCED_FACE('',(#2731),#711,.T.) ;
#27467=ADVANCED_FACE('',(#2732),#712,.T.) ;
#27468=ADVANCED_FACE('',(#2733),#713,.T.) ;
#27469=ADVANCED_FACE('',(#2734),#714,.T.) ;
#27470=ADVANCED_FACE('',(#2735),#715,.T.) ;
#27471=ADVANCED_FACE('',(#2736),#716,.T.) ;
#27472=ADVANCED_FACE('',(#2737),#717,.T.) ;
#27473=ADVANCED_FACE('',(#2738),#718,.T.) ;
#27474=ADVANCED_FACE('',(#2739),#719,.T.) ;
#27475=ADVANCED_FACE('',(#2740),#720,.T.) ;
#27476=ADVANCED_FACE('',(#2741),#721,.T.) ;
#27477=ADVANCED_FACE('',(#2742),#722,.T.) ;
#27478=ADVANCED_FACE('',(#2743),#723,.T.) ;
#27479=ADVANCED_FACE('',(#2744),#724,.T.) ;
#27480=ADVANCED_FACE('',(#2745),#725,.T.) ;
#27481=ADVANCED_FACE('',(#2746),#726,.T.) ;
#27482=ADVANCED_FACE('',(#2747),#26707,.T.) ;
#27483=ADVANCED_FACE('',(#2748),#26708,.T.) ;
#27484=ADVANCED_FACE('',(#2749),#26709,.T.) ;
#27485=ADVANCED_FACE('',(#2750),#26710,.T.) ;
#27486=ADVANCED_FACE('',(#2751),#26711,.T.) ;
#27487=ADVANCED_FACE('',(#2752),#26712,.T.) ;
#27488=ADVANCED_FACE('',(#2753),#26713,.T.) ;
#27489=ADVANCED_FACE('',(#2754),#26714,.T.) ;
#27490=ADVANCED_FACE('',(#2755),#26715,.T.) ;
#27491=ADVANCED_FACE('',(#2756),#26716,.T.) ;
#27492=ADVANCED_FACE('',(#2757),#26717,.T.) ;
#27493=ADVANCED_FACE('',(#2758),#26718,.T.) ;
#27494=ADVANCED_FACE('',(#2759),#26719,.T.) ;
#27495=ADVANCED_FACE('',(#2760),#26720,.T.) ;
#27496=ADVANCED_FACE('',(#2761),#26721,.T.) ;
#27497=ADVANCED_FACE('',(#2762),#26722,.T.) ;
#27498=ADVANCED_FACE('',(#2763),#26723,.T.) ;
#27499=ADVANCED_FACE('',(#2764),#26724,.T.) ;
#27500=ADVANCED_FACE('',(#2765),#26725,.T.) ;
#27501=ADVANCED_FACE('',(#2766),#26726,.T.) ;
#27502=ADVANCED_FACE('',(#2767),#26727,.T.) ;
#27503=ADVANCED_FACE('',(#2768),#26728,.T.) ;
#27504=ADVANCED_FACE('',(#2769),#26729,.T.) ;
#27505=ADVANCED_FACE('',(#2770),#26730,.T.) ;
#27506=ADVANCED_FACE('',(#2771),#26731,.T.) ;
#27507=ADVANCED_FACE('',(#2772),#26732,.T.) ;
#27508=ADVANCED_FACE('',(#2773),#26733,.T.) ;
#27509=ADVANCED_FACE('',(#2774),#26734,.T.) ;
#28633=CLOSED_SHELL('',(#27454,#27455,#27456,#27457,#27458,#27459,#27460,
#27461,#27462,#27463,#27464,#27465,#27466,#27467,#27468,#27469,#27470,#27471,
#27472,#27473,#27474,#27475,#27476,#27477,#27478,#27479,#27480,#27481,#27482,
#27483,#27484,#27485,#27486,#27487,#27488,#27489,#27490,#27491,#27492,#27493,
#27494,#27495,#27496,#27497,#27498,#27499,#27500,#27501,#27502,#27503,#27504,
#27505,#27506,#27507,#27508,#27509)) ;
#29730=AXIS2_PLACEMENT_3D('',#43441,#34360,#34361) ;
#29731=AXIS2_PLACEMENT_3D('',#43442,#34362,#34363) ;
#29732=AXIS2_PLACEMENT_3D('',#43445,#34364,#34365) ;
#29733=AXIS2_PLACEMENT_3D('',#43446,#34366,#34367) ;
#29734=AXIS2_PLACEMENT_3D('',#43447,#34368,#34369) ;
#29735=AXIS2_PLACEMENT_3D('',#43450,#34370,#34371) ;
#29736=AXIS2_PLACEMENT_3D('',#43451,#34372,#34373) ;
#29737=AXIS2_PLACEMENT_3D('',#43452,#34374,#34375) ;
#29738=AXIS2_PLACEMENT_3D('',#43455,#34376,#34377) ;
#29739=AXIS2_PLACEMENT_3D('',#43456,#34378,#34379) ;
#29740=AXIS2_PLACEMENT_3D('',#43457,#34380,#34381) ;
#29741=AXIS2_PLACEMENT_3D('',#43460,#34382,#34383) ;
#29742=AXIS2_PLACEMENT_3D('',#43461,#34384,#34385) ;
#29743=AXIS2_PLACEMENT_3D('',#43462,#34386,#34387) ;
#29744=AXIS2_PLACEMENT_3D('',#43465,#34388,#34389) ;
#29745=AXIS2_PLACEMENT_3D('',#43466,#34390,#34391) ;
#29746=AXIS2_PLACEMENT_3D('',#43467,#34392,#34393) ;
#29747=AXIS2_PLACEMENT_3D('',#43470,#34394,#34395) ;
#29748=AXIS2_PLACEMENT_3D('',#43471,#34396,#34397) ;
#29749=AXIS2_PLACEMENT_3D('',#43472,#34398,#34399) ;
#29750=AXIS2_PLACEMENT_3D('',#43475,#34400,#34401) ;
#29751=AXIS2_PLACEMENT_3D('',#43476,#34402,#34403) ;
#29752=AXIS2_PLACEMENT_3D('',#43477,#34404,#34405) ;
#29753=AXIS2_PLACEMENT_3D('',#43480,#34406,#34407) ;
#29754=AXIS2_PLACEMENT_3D('',#43482,#34408,#34409) ;
#29755=AXIS2_PLACEMENT_3D('',#43483,#34410,#34411) ;
#29756=AXIS2_PLACEMENT_3D('',#43484,#34412,#34413) ;
#29757=AXIS2_PLACEMENT_3D('',#43487,#34414,#34415) ;
#29758=AXIS2_PLACEMENT_3D('',#43489,#34416,#34417) ;
#29759=AXIS2_PLACEMENT_3D('',#43491,#34418,#34419) ;
#29760=AXIS2_PLACEMENT_3D('',#43492,#34420,#34421) ;
#29761=AXIS2_PLACEMENT_3D('',#43493,#34422,#34423) ;
#29762=AXIS2_PLACEMENT_3D('',#43496,#34424,#34425) ;
#29763=AXIS2_PLACEMENT_3D('',#43498,#34426,#34427) ;
#29764=AXIS2_PLACEMENT_3D('',#43500,#34428,#34429) ;
#29765=AXIS2_PLACEMENT_3D('',#43501,#34430,#34431) ;
#29766=AXIS2_PLACEMENT_3D('',#43502,#34432,#34433) ;
#29767=AXIS2_PLACEMENT_3D('',#43505,#34434,#34435) ;
#29768=AXIS2_PLACEMENT_3D('',#43507,#34436,#34437) ;
#29769=AXIS2_PLACEMENT_3D('',#43509,#34438,#34439) ;
#29770=AXIS2_PLACEMENT_3D('',#43510,#34440,#34441) ;
#29771=AXIS2_PLACEMENT_3D('',#43511,#34442,#34443) ;
#29772=AXIS2_PLACEMENT_3D('',#43514,#34444,#34445) ;
#29773=AXIS2_PLACEMENT_3D('',#43516,#34446,#34447) ;
#29774=AXIS2_PLACEMENT_3D('',#43518,#34448,#34449) ;
#29775=AXIS2_PLACEMENT_3D('',#43519,#34450,#34451) ;
#29776=AXIS2_PLACEMENT_3D('',#43520,#34452,#34453) ;
#29777=AXIS2_PLACEMENT_3D('',#43523,#34454,#34455) ;
#29778=AXIS2_PLACEMENT_3D('',#43525,#34456,#34457) ;
#29779=AXIS2_PLACEMENT_3D('',#43527,#34458,#34459) ;
#29780=AXIS2_PLACEMENT_3D('',#43528,#34460,#34461) ;
#29781=AXIS2_PLACEMENT_3D('',#43529,#34462,#34463) ;
#29782=AXIS2_PLACEMENT_3D('',#43532,#34464,#34465) ;
#29783=AXIS2_PLACEMENT_3D('',#43534,#34466,#34467) ;
#29784=AXIS2_PLACEMENT_3D('',#43536,#34468,#34469) ;
#29785=AXIS2_PLACEMENT_3D('',#43537,#34470,#34471) ;
#29786=AXIS2_PLACEMENT_3D('',#43538,#34472,#34473) ;
#29787=AXIS2_PLACEMENT_3D('',#43541,#34474,#34475) ;
#29788=AXIS2_PLACEMENT_3D('',#43543,#34476,#34477) ;
#29789=AXIS2_PLACEMENT_3D('',#43545,#34478,#34479) ;
#29790=AXIS2_PLACEMENT_3D('',#43546,#34480,#34481) ;
#29791=AXIS2_PLACEMENT_3D('',#43547,#34482,#34483) ;
#29792=AXIS2_PLACEMENT_3D('',#43550,#34484,#34485) ;
#29793=AXIS2_PLACEMENT_3D('',#43552,#34486,#34487) ;
#29794=AXIS2_PLACEMENT_3D('',#43554,#34488,#34489) ;
#29795=AXIS2_PLACEMENT_3D('',#43555,#34490,#34491) ;
#29796=AXIS2_PLACEMENT_3D('',#43556,#34492,#34493) ;
#29797=AXIS2_PLACEMENT_3D('',#43559,#34494,#34495) ;
#29798=AXIS2_PLACEMENT_3D('',#43561,#34496,#34497) ;
#29799=AXIS2_PLACEMENT_3D('',#43563,#34498,#34499) ;
#29800=AXIS2_PLACEMENT_3D('',#43564,#34500,#34501) ;
#29801=AXIS2_PLACEMENT_3D('',#43565,#34502,#34503) ;
#29802=AXIS2_PLACEMENT_3D('',#43568,#34504,#34505) ;
#29803=AXIS2_PLACEMENT_3D('',#43570,#34506,#34507) ;
#29804=AXIS2_PLACEMENT_3D('',#43572,#34508,#34509) ;
#29805=AXIS2_PLACEMENT_3D('',#43573,#34510,#34511) ;
#29806=AXIS2_PLACEMENT_3D('',#43574,#34512,#34513) ;
#29807=AXIS2_PLACEMENT_3D('',#43577,#34514,#34515) ;
#29808=AXIS2_PLACEMENT_3D('',#43579,#34516,#34517) ;
#29809=AXIS2_PLACEMENT_3D('',#43581,#34518,#34519) ;
#29810=AXIS2_PLACEMENT_3D('',#43582,#34520,#34521) ;
#29811=AXIS2_PLACEMENT_3D('',#43583,#34522,#34523) ;
#29812=AXIS2_PLACEMENT_3D('',#43586,#34524,#34525) ;
#29813=AXIS2_PLACEMENT_3D('',#43588,#34526,#34527) ;
#29814=AXIS2_PLACEMENT_3D('',#43590,#34528,#34529) ;
#29815=AXIS2_PLACEMENT_3D('',#43591,#34530,#34531) ;
#29816=AXIS2_PLACEMENT_3D('',#43592,#34532,#34533) ;
#29817=AXIS2_PLACEMENT_3D('',#43595,#34534,#34535) ;
#29818=AXIS2_PLACEMENT_3D('',#43597,#34536,#34537) ;
#29819=AXIS2_PLACEMENT_3D('',#43599,#34538,#34539) ;
#29820=AXIS2_PLACEMENT_3D('',#43600,#34540,#34541) ;
#29821=AXIS2_PLACEMENT_3D('',#43601,#34542,#34543) ;
#29822=AXIS2_PLACEMENT_3D('',#43604,#34544,#34545) ;
#29823=AXIS2_PLACEMENT_3D('',#43606,#34546,#34547) ;
#29824=AXIS2_PLACEMENT_3D('',#43607,#34548,#34549) ;
#29825=AXIS2_PLACEMENT_3D('',#43608,#34550,#34551) ;
#29826=AXIS2_PLACEMENT_3D('',#43611,#34552,#34553) ;
#29827=AXIS2_PLACEMENT_3D('',#43612,#34554,#34555) ;
#29828=AXIS2_PLACEMENT_3D('',#43613,#34556,#34557) ;
#29829=AXIS2_PLACEMENT_3D('',#43616,#34558,#34559) ;
#29830=AXIS2_PLACEMENT_3D('',#43617,#34560,#34561) ;
#29831=AXIS2_PLACEMENT_3D('',#43618,#34562,#34563) ;
#29832=AXIS2_PLACEMENT_3D('',#43621,#34564,#34565) ;
#29833=AXIS2_PLACEMENT_3D('',#43622,#34566,#34567) ;
#29834=AXIS2_PLACEMENT_3D('',#43623,#34568,#34569) ;
#29835=AXIS2_PLACEMENT_3D('',#43626,#34570,#34571) ;
#29836=AXIS2_PLACEMENT_3D('',#43627,#34572,#34573) ;
#29837=AXIS2_PLACEMENT_3D('',#43628,#34574,#34575) ;
#29838=AXIS2_PLACEMENT_3D('',#43631,#34576,#34577) ;
#29839=AXIS2_PLACEMENT_3D('',#43632,#34578,#34579) ;
#29840=AXIS2_PLACEMENT_3D('',#43633,#34580,#34581) ;
#29841=AXIS2_PLACEMENT_3D('',#43636,#34582,#34583) ;
#29842=AXIS2_PLACEMENT_3D('',#43637,#34584,#34585) ;
#29843=AXIS2_PLACEMENT_3D('',#43638,#34586,#34587) ;
#29844=AXIS2_PLACEMENT_3D('',#43640,#34588,#34589) ;
#29845=AXIS2_PLACEMENT_3D('',#43641,#34590,#34591) ;
#29846=AXIS2_PLACEMENT_3D('',#43644,#34593,#34594) ;
#29847=AXIS2_PLACEMENT_3D('',#43645,#34595,#34596) ;
#29848=AXIS2_PLACEMENT_3D('',#43646,#34597,#34598) ;
#29849=AXIS2_PLACEMENT_3D('',#43649,#34600,#34601) ;
#29850=AXIS2_PLACEMENT_3D('',#43650,#34602,#34603) ;
#29851=AXIS2_PLACEMENT_3D('',#43651,#34604,#34605) ;
#29852=AXIS2_PLACEMENT_3D('',#43654,#34607,#34608) ;
#29853=AXIS2_PLACEMENT_3D('',#43655,#34609,#34610) ;
#29854=AXIS2_PLACEMENT_3D('',#43656,#34611,#34612) ;
#29855=AXIS2_PLACEMENT_3D('',#43659,#34614,#34615) ;
#29856=AXIS2_PLACEMENT_3D('',#43660,#34616,#34617) ;
#29857=AXIS2_PLACEMENT_3D('',#43661,#34618,#34619) ;
#29858=AXIS2_PLACEMENT_3D('',#43664,#34621,#34622) ;
#29859=AXIS2_PLACEMENT_3D('',#43665,#34623,#34624) ;
#29860=AXIS2_PLACEMENT_3D('',#43666,#34625,#34626) ;
#29861=AXIS2_PLACEMENT_3D('',#43669,#34628,#34629) ;
#29862=AXIS2_PLACEMENT_3D('',#43670,#34630,#34631) ;
#29863=AXIS2_PLACEMENT_3D('',#43671,#34632,#34633) ;
#29864=AXIS2_PLACEMENT_3D('',#43674,#34635,#34636) ;
#29865=AXIS2_PLACEMENT_3D('',#43675,#34637,#34638) ;
#29866=AXIS2_PLACEMENT_3D('',#43676,#34639,#34640) ;
#29867=AXIS2_PLACEMENT_3D('',#43678,#34642,#34643) ;
#29868=AXIS2_PLACEMENT_3D('',#43679,#34644,#34645) ;
#29869=AXIS2_PLACEMENT_3D('',#43681,#34647,#34648) ;
#29870=AXIS2_PLACEMENT_3D('',#43682,#34649,#34650) ;
#29871=AXIS2_PLACEMENT_3D('',#43684,#34652,#34653) ;
#29872=AXIS2_PLACEMENT_3D('',#43685,#34654,#34655) ;
#29873=AXIS2_PLACEMENT_3D('',#43687,#34657,#34658) ;
#29874=AXIS2_PLACEMENT_3D('',#43688,#34659,#34660) ;
#29875=AXIS2_PLACEMENT_3D('',#43690,#34662,#34663) ;
#29876=AXIS2_PLACEMENT_3D('',#43691,#34664,#34665) ;
#29877=AXIS2_PLACEMENT_3D('',#43693,#34667,#34668) ;
#29878=AXIS2_PLACEMENT_3D('',#43694,#34669,#34670) ;
#29879=AXIS2_PLACEMENT_3D('',#43696,#34672,#34673) ;
#29880=AXIS2_PLACEMENT_3D('',#43697,#34674,#34675) ;
#29881=AXIS2_PLACEMENT_3D('',#43699,#34677,#34678) ;
#29882=AXIS2_PLACEMENT_3D('',#43700,#34679,#34680) ;
#29883=AXIS2_PLACEMENT_3D('',#43702,#34682,#34683) ;
#29884=AXIS2_PLACEMENT_3D('',#43703,#34684,#34685) ;
#29885=AXIS2_PLACEMENT_3D('',#43705,#34687,#34688) ;
#29886=AXIS2_PLACEMENT_3D('',#43706,#34689,#34690) ;
#29887=AXIS2_PLACEMENT_3D('',#43708,#34692,#34693) ;
#29888=AXIS2_PLACEMENT_3D('',#43709,#34694,#34695) ;
#29889=AXIS2_PLACEMENT_3D('',#43711,#34697,#34698) ;
#29890=AXIS2_PLACEMENT_3D('',#43712,#34699,#34700) ;
#29891=AXIS2_PLACEMENT_3D('',#43714,#34702,#34703) ;
#29892=AXIS2_PLACEMENT_3D('',#43715,#34704,#34705) ;
#29893=AXIS2_PLACEMENT_3D('',#43718,#34707,#34708) ;
#29894=AXIS2_PLACEMENT_3D('',#43719,#34709,#34710) ;
#29895=AXIS2_PLACEMENT_3D('',#43720,#34711,#34712) ;
#29896=AXIS2_PLACEMENT_3D('',#43723,#34714,#34715) ;
#29897=AXIS2_PLACEMENT_3D('',#43724,#34716,#34717) ;
#29898=AXIS2_PLACEMENT_3D('',#43725,#34718,#34719) ;
#29899=AXIS2_PLACEMENT_3D('',#43728,#34721,#34722) ;
#29900=AXIS2_PLACEMENT_3D('',#43729,#34723,#34724) ;
#29901=AXIS2_PLACEMENT_3D('',#43730,#34725,#34726) ;
#29902=AXIS2_PLACEMENT_3D('',#43733,#34728,#34729) ;
#29903=AXIS2_PLACEMENT_3D('',#43734,#34730,#34731) ;
#29904=AXIS2_PLACEMENT_3D('',#43735,#34732,#34733) ;
#29905=AXIS2_PLACEMENT_3D('',#43738,#34735,#34736) ;
#29906=AXIS2_PLACEMENT_3D('',#43739,#34737,#34738) ;
#29907=AXIS2_PLACEMENT_3D('',#43740,#34739,#34740) ;
#29908=AXIS2_PLACEMENT_3D('',#43743,#34742,#34743) ;
#29909=AXIS2_PLACEMENT_3D('',#43744,#34744,#34745) ;
#29910=AXIS2_PLACEMENT_3D('',#43745,#34746,#34747) ;
#29911=AXIS2_PLACEMENT_3D('',#43748,#34749,#34750) ;
#29912=AXIS2_PLACEMENT_3D('',#43749,#34751,#34752) ;
#29913=AXIS2_PLACEMENT_3D('',#43750,#34753,#34754) ;
#34360=DIRECTION('axis',(0.,0.,1.)) ;
#34361=DIRECTION('refdir',(1.,0.,0.)) ;
#34362=DIRECTION('center_axis',(0.,0.,1.)) ;
#34363=DIRECTION('ref_axis',(1.,0.,0.)) ;
#34364=DIRECTION('center_axis',(0.111964476103308,0.993712209893243,0.)) ;
#34365=DIRECTION('ref_axis',(0.993712209893243,-0.111964476103308,0.)) ;
#34366=DIRECTION('center_axis',(0.111964476103307,-0.993712209893243,0.)) ;
#34367=DIRECTION('ref_axis',(0.993712209893243,0.111964476103307,0.)) ;
#34368=DIRECTION('center_axis',(0.,0.,1.)) ;
#34369=DIRECTION('ref_axis',(1.,0.,0.)) ;
#34370=DIRECTION('center_axis',(-0.111964476103308,-0.993712209893243,0.)) ;
#34371=DIRECTION('ref_axis',(0.993712209893243,-0.111964476103308,0.)) ;
#34372=DIRECTION('center_axis',(0.330279061955167,0.943883330308368,0.)) ;
#34373=DIRECTION('ref_axis',(0.943883330308368,-0.330279061955167,0.)) ;
#34374=DIRECTION('center_axis',(0.,0.,1.)) ;
#34375=DIRECTION('ref_axis',(1.,0.,0.)) ;
#34376=DIRECTION('center_axis',(-0.330279061955167,-0.943883330308368,0.)) ;
#34377=DIRECTION('ref_axis',(0.943883330308368,-0.330279061955167,0.)) ;
#34378=DIRECTION('center_axis',(0.532032076515336,0.846724199228284,0.)) ;
#34379=DIRECTION('ref_axis',(0.846724199228285,-0.532032076515336,0.)) ;
#34380=DIRECTION('center_axis',(0.,0.,1.)) ;
#34381=DIRECTION('ref_axis',(1.,0.,0.)) ;
#34382=DIRECTION('center_axis',(-0.532032076515336,-0.846724199228284,0.)) ;
#34383=DIRECTION('ref_axis',(0.846724199228285,-0.532032076515336,0.)) ;
#34384=DIRECTION('center_axis',(0.707106781186548,0.707106781186547,0.)) ;
#34385=DIRECTION('ref_axis',(0.707106781186547,-0.707106781186548,0.)) ;
#34386=DIRECTION('center_axis',(0.,0.,1.)) ;
#34387=DIRECTION('ref_axis',(1.,0.,0.)) ;
#34388=DIRECTION('center_axis',(-0.707106781186548,-0.707106781186547,0.)) ;
#34389=DIRECTION('ref_axis',(0.707106781186547,-0.707106781186548,0.)) ;
#34390=DIRECTION('center_axis',(0.846724199228284,0.532032076515337,0.)) ;
#34391=DIRECTION('ref_axis',(0.532032076515337,-0.846724199228284,0.)) ;
#34392=DIRECTION('center_axis',(0.,0.,1.)) ;
#34393=DIRECTION('ref_axis',(1.,0.,0.)) ;
#34394=DIRECTION('center_axis',(-0.846724199228284,-0.532032076515337,0.)) ;
#34395=DIRECTION('ref_axis',(0.532032076515337,-0.846724199228284,0.)) ;
#34396=DIRECTION('center_axis',(0.943883330308368,0.330279061955166,0.)) ;
#34397=DIRECTION('ref_axis',(0.330279061955166,-0.943883330308368,0.)) ;
#34398=DIRECTION('center_axis',(0.,0.,1.)) ;
#34399=DIRECTION('ref_axis',(1.,0.,0.)) ;
#34400=DIRECTION('center_axis',(-0.943883330308368,-0.330279061955166,0.)) ;
#34401=DIRECTION('ref_axis',(0.330279061955166,-0.943883330308368,0.)) ;
#34402=DIRECTION('center_axis',(0.993712209893243,0.111964476103307,0.)) ;
#34403=DIRECTION('ref_axis',(0.111964476103307,-0.993712209893243,0.)) ;
#34404=DIRECTION('center_axis',(6.12323399573676E-17,0.,1.)) ;
#34405=DIRECTION('ref_axis',(1.,0.,0.)) ;
#34406=DIRECTION('center_axis',(-0.993712209893243,-0.111964476103307,0.)) ;
#34407=DIRECTION('ref_axis',(0.111964476103307,-0.993712209893243,0.)) ;
#34408=DIRECTION('center_axis',(0.993712209893243,-0.111964476103307,0.)) ;
#34409=DIRECTION('ref_axis',(0.111964476103307,0.993712209893243,0.)) ;
#34410=DIRECTION('center_axis',(0.993712209893243,-0.111964476103307,0.)) ;
#34411=DIRECTION('ref_axis',(0.111964476103307,0.993712209893243,0.)) ;
#34412=DIRECTION('center_axis',(0.,0.,1.)) ;
#34413=DIRECTION('ref_axis',(1.,0.,0.)) ;
#34414=DIRECTION('center_axis',(-0.993712209893243,0.111964476103307,0.)) ;
#34415=DIRECTION('ref_axis',(0.111964476103307,0.993712209893243,0.)) ;
#34416=DIRECTION('center_axis',(-0.993712209893243,0.111964476103307,0.)) ;
#34417=DIRECTION('ref_axis',(0.111964476103307,0.993712209893243,0.)) ;
#34418=DIRECTION('center_axis',(0.943883330308367,-0.330279061955168,0.)) ;
#34419=DIRECTION('ref_axis',(0.330279061955168,0.943883330308367,0.)) ;
#34420=DIRECTION('center_axis',(0.943883330308367,-0.330279061955168,0.)) ;
#34421=DIRECTION('ref_axis',(0.330279061955168,0.943883330308367,0.)) ;
#34422=DIRECTION('center_axis',(0.,0.,1.)) ;
#34423=DIRECTION('ref_axis',(1.,0.,0.)) ;
#34424=DIRECTION('center_axis',(-0.943883330308367,0.330279061955168,0.)) ;
#34425=DIRECTION('ref_axis',(0.330279061955168,0.943883330308367,0.)) ;
#34426=DIRECTION('center_axis',(-0.943883330308367,0.330279061955168,0.)) ;
#34427=DIRECTION('ref_axis',(0.330279061955168,0.943883330308367,0.)) ;
#34428=DIRECTION('center_axis',(0.846724199228284,-0.532032076515337,0.)) ;
#34429=DIRECTION('ref_axis',(0.532032076515337,0.846724199228284,0.)) ;
#34430=DIRECTION('center_axis',(0.846724199228284,-0.532032076515337,0.)) ;
#34431=DIRECTION('ref_axis',(0.532032076515337,0.846724199228284,0.)) ;
#34432=DIRECTION('center_axis',(0.,0.,1.)) ;
#34433=DIRECTION('ref_axis',(1.,0.,0.)) ;
#34434=DIRECTION('center_axis',(-0.846724199228284,0.532032076515337,0.)) ;
#34435=DIRECTION('ref_axis',(0.532032076515337,0.846724199228284,0.)) ;
#34436=DIRECTION('center_axis',(-0.846724199228284,0.532032076515337,0.)) ;
#34437=DIRECTION('ref_axis',(0.532032076515337,0.846724199228284,0.)) ;
#34438=DIRECTION('center_axis',(0.707106781186548,-0.707106781186547,0.)) ;
#34439=DIRECTION('ref_axis',(0.707106781186547,0.707106781186548,0.)) ;
#34440=DIRECTION('center_axis',(0.707106781186548,-0.707106781186547,0.)) ;
#34441=DIRECTION('ref_axis',(0.707106781186547,0.707106781186548,0.)) ;
#34442=DIRECTION('center_axis',(0.,0.,1.)) ;
#34443=DIRECTION('ref_axis',(1.,0.,0.)) ;
#34444=DIRECTION('center_axis',(-0.707106781186548,0.707106781186547,0.)) ;
#34445=DIRECTION('ref_axis',(0.707106781186547,0.707106781186548,0.)) ;
#34446=DIRECTION('center_axis',(-0.707106781186548,0.707106781186547,0.)) ;
#34447=DIRECTION('ref_axis',(0.707106781186547,0.707106781186548,0.)) ;
#34448=DIRECTION('center_axis',(0.532032076515336,-0.846724199228284,0.)) ;
#34449=DIRECTION('ref_axis',(0.846724199228284,0.532032076515336,0.)) ;
#34450=DIRECTION('center_axis',(0.532032076515336,-0.846724199228284,0.)) ;
#34451=DIRECTION('ref_axis',(0.846724199228284,0.532032076515336,0.)) ;
#34452=DIRECTION('center_axis',(0.,0.,1.)) ;
#34453=DIRECTION('ref_axis',(1.,0.,0.)) ;
#34454=DIRECTION('center_axis',(-0.532032076515336,0.846724199228284,0.)) ;
#34455=DIRECTION('ref_axis',(0.846724199228284,0.532032076515336,0.)) ;
#34456=DIRECTION('center_axis',(-0.532032076515336,0.846724199228284,0.)) ;
#34457=DIRECTION('ref_axis',(0.846724199228284,0.532032076515336,0.)) ;
#34458=DIRECTION('center_axis',(0.330279061955167,-0.943883330308368,0.)) ;
#34459=DIRECTION('ref_axis',(0.943883330308368,0.330279061955167,0.)) ;
#34460=DIRECTION('center_axis',(0.330279061955167,-0.943883330308368,0.)) ;
#34461=DIRECTION('ref_axis',(0.943883330308368,0.330279061955167,0.)) ;
#34462=DIRECTION('center_axis',(0.,0.,1.)) ;
#34463=DIRECTION('ref_axis',(1.,0.,0.)) ;
#34464=DIRECTION('center_axis',(-0.330279061955167,0.943883330308368,0.)) ;
#34465=DIRECTION('ref_axis',(0.943883330308368,0.330279061955167,0.)) ;
#34466=DIRECTION('center_axis',(-0.330279061955167,0.943883330308368,0.)) ;
#34467=DIRECTION('ref_axis',(0.943883330308368,0.330279061955167,0.)) ;
#34468=DIRECTION('center_axis',(0.111964476103307,-0.993712209893243,0.)) ;
#34469=DIRECTION('ref_axis',(0.993712209893243,0.111964476103307,0.)) ;
#34470=DIRECTION('center_axis',(0.111964476103307,-0.993712209893243,0.)) ;
#34471=DIRECTION('ref_axis',(0.993712209893243,0.111964476103307,0.)) ;
#34472=DIRECTION('center_axis',(0.,-1.32134201624519E-28,1.)) ;
#34473=DIRECTION('ref_axis',(-1.,-2.15839602455122E-12,0.)) ;
#34474=DIRECTION('center_axis',(-0.111964476103307,0.993712209893243,0.)) ;
#34475=DIRECTION('ref_axis',(0.993712209893243,0.111964476103307,0.)) ;
#34476=DIRECTION('center_axis',(-0.111964476103307,0.993712209893243,0.)) ;
#34477=DIRECTION('ref_axis',(0.993712209893243,0.111964476103307,0.)) ;
#34478=DIRECTION('center_axis',(-0.111964476103307,-0.993712209893243,0.)) ;
#34479=DIRECTION('ref_axis',(0.993712209893243,-0.111964476103307,0.)) ;
#34480=DIRECTION('center_axis',(-0.111964476103307,-0.993712209893243,0.)) ;
#34481=DIRECTION('ref_axis',(0.993712209893243,-0.111964476103307,0.)) ;
#34482=DIRECTION('center_axis',(0.,0.,1.)) ;
#34483=DIRECTION('ref_axis',(1.,0.,0.)) ;
#34484=DIRECTION('center_axis',(0.111964476103307,0.993712209893243,0.)) ;
#34485=DIRECTION('ref_axis',(0.993712209893243,-0.111964476103307,0.)) ;
#34486=DIRECTION('center_axis',(0.111964476103307,0.993712209893243,0.)) ;
#34487=DIRECTION('ref_axis',(0.993712209893243,-0.111964476103307,0.)) ;
#34488=DIRECTION('center_axis',(-0.330279061955167,-0.943883330308367,0.)) ;
#34489=DIRECTION('ref_axis',(0.943883330308368,-0.330279061955167,0.)) ;
#34490=DIRECTION('center_axis',(-0.330279061955167,-0.943883330308367,0.)) ;
#34491=DIRECTION('ref_axis',(0.943883330308368,-0.330279061955167,0.)) ;
#34492=DIRECTION('center_axis',(0.,0.,1.)) ;
#34493=DIRECTION('ref_axis',(1.,0.,0.)) ;
#34494=DIRECTION('center_axis',(0.330279061955167,0.943883330308367,0.)) ;
#34495=DIRECTION('ref_axis',(0.943883330308368,-0.330279061955167,0.)) ;
#34496=DIRECTION('center_axis',(0.330279061955167,0.943883330308367,0.)) ;
#34497=DIRECTION('ref_axis',(0.943883330308368,-0.330279061955167,0.)) ;
#34498=DIRECTION('center_axis',(-0.532032076515337,-0.846724199228284,0.)) ;
#34499=DIRECTION('ref_axis',(0.846724199228284,-0.532032076515337,0.)) ;
#34500=DIRECTION('center_axis',(-0.532032076515337,-0.846724199228284,0.)) ;
#34501=DIRECTION('ref_axis',(0.846724199228284,-0.532032076515337,0.)) ;
#34502=DIRECTION('center_axis',(0.,0.,1.)) ;
#34503=DIRECTION('ref_axis',(1.,0.,0.)) ;
#34504=DIRECTION('center_axis',(0.532032076515337,0.846724199228284,0.)) ;
#34505=DIRECTION('ref_axis',(0.846724199228284,-0.532032076515337,0.)) ;
#34506=DIRECTION('center_axis',(0.532032076515337,0.846724199228284,0.)) ;
#34507=DIRECTION('ref_axis',(0.846724199228284,-0.532032076515337,0.)) ;
#34508=DIRECTION('center_axis',(-0.707106781186548,-0.707106781186548,0.)) ;
#34509=DIRECTION('ref_axis',(0.707106781186548,-0.707106781186548,0.)) ;
#34510=DIRECTION('center_axis',(-0.707106781186548,-0.707106781186548,0.)) ;
#34511=DIRECTION('ref_axis',(0.707106781186548,-0.707106781186548,0.)) ;
#34512=DIRECTION('center_axis',(0.,0.,1.)) ;
#34513=DIRECTION('ref_axis',(1.,0.,0.)) ;
#34514=DIRECTION('center_axis',(0.707106781186548,0.707106781186548,0.)) ;
#34515=DIRECTION('ref_axis',(0.707106781186548,-0.707106781186548,0.)) ;
#34516=DIRECTION('center_axis',(0.707106781186548,0.707106781186548,0.)) ;
#34517=DIRECTION('ref_axis',(0.707106781186548,-0.707106781186548,0.)) ;
#34518=DIRECTION('center_axis',(-0.846724199228285,-0.532032076515336,0.)) ;
#34519=DIRECTION('ref_axis',(0.532032076515336,-0.846724199228285,0.)) ;
#34520=DIRECTION('center_axis',(-0.846724199228285,-0.532032076515336,0.)) ;
#34521=DIRECTION('ref_axis',(0.532032076515336,-0.846724199228285,0.)) ;
#34522=DIRECTION('center_axis',(0.,0.,1.)) ;
#34523=DIRECTION('ref_axis',(1.,0.,0.)) ;
#34524=DIRECTION('center_axis',(0.846724199228285,0.532032076515336,0.)) ;
#34525=DIRECTION('ref_axis',(0.532032076515336,-0.846724199228285,0.)) ;
#34526=DIRECTION('center_axis',(0.846724199228285,0.532032076515336,0.)) ;
#34527=DIRECTION('ref_axis',(0.532032076515336,-0.846724199228285,0.)) ;
#34528=DIRECTION('center_axis',(-0.943883330308367,-0.330279061955168,0.)) ;
#34529=DIRECTION('ref_axis',(0.330279061955168,-0.943883330308367,0.)) ;
#34530=DIRECTION('center_axis',(-0.943883330308367,-0.330279061955168,0.)) ;
#34531=DIRECTION('ref_axis',(0.330279061955168,-0.943883330308367,0.)) ;
#34532=DIRECTION('center_axis',(0.,0.,1.)) ;
#34533=DIRECTION('ref_axis',(1.,0.,0.)) ;
#34534=DIRECTION('center_axis',(0.943883330308367,0.330279061955168,0.)) ;
#34535=DIRECTION('ref_axis',(0.330279061955168,-0.943883330308367,0.)) ;
#34536=DIRECTION('center_axis',(0.943883330308367,0.330279061955168,0.)) ;
#34537=DIRECTION('ref_axis',(0.330279061955168,-0.943883330308367,0.)) ;
#34538=DIRECTION('center_axis',(-0.993712209893243,-0.111964476103307,0.)) ;
#34539=DIRECTION('ref_axis',(0.111964476103307,-0.993712209893243,0.)) ;
#34540=DIRECTION('center_axis',(-0.993712209893243,-0.111964476103307,0.)) ;
#34541=DIRECTION('ref_axis',(0.111964476103307,-0.993712209893243,0.)) ;
#34542=DIRECTION('center_axis',(6.12323399573676E-17,0.,1.)) ;
#34543=DIRECTION('ref_axis',(1.,0.,0.)) ;
#34544=DIRECTION('center_axis',(0.993712209893243,0.111964476103307,0.)) ;
#34545=DIRECTION('ref_axis',(0.111964476103307,-0.993712209893243,0.)) ;
#34546=DIRECTION('center_axis',(0.993712209893243,0.111964476103307,0.)) ;
#34547=DIRECTION('ref_axis',(0.111964476103307,-0.993712209893243,0.)) ;
#34548=DIRECTION('center_axis',(-0.993712209893243,0.111964476103307,0.)) ;
#34549=DIRECTION('ref_axis',(0.111964476103307,0.993712209893243,0.)) ;
#34550=DIRECTION('center_axis',(0.,0.,1.)) ;
#34551=DIRECTION('ref_axis',(1.,0.,0.)) ;
#34552=DIRECTION('center_axis',(0.993712209893243,-0.111964476103307,0.)) ;
#34553=DIRECTION('ref_axis',(0.111964476103307,0.993712209893243,0.)) ;
#34554=DIRECTION('center_axis',(-0.943883330308367,0.330279061955168,0.)) ;
#34555=DIRECTION('ref_axis',(0.330279061955168,0.943883330308367,0.)) ;
#34556=DIRECTION('center_axis',(0.,0.,1.)) ;
#34557=DIRECTION('ref_axis',(1.,0.,0.)) ;
#34558=DIRECTION('center_axis',(0.943883330308367,-0.330279061955168,0.)) ;
#34559=DIRECTION('ref_axis',(0.330279061955168,0.943883330308367,0.)) ;
#34560=DIRECTION('center_axis',(-0.846724199228284,0.532032076515336,0.)) ;
#34561=DIRECTION('ref_axis',(0.532032076515336,0.846724199228284,0.)) ;
#34562=DIRECTION('center_axis',(0.,0.,1.)) ;
#34563=DIRECTION('ref_axis',(1.,0.,0.)) ;
#34564=DIRECTION('center_axis',(0.846724199228284,-0.532032076515336,0.)) ;
#34565=DIRECTION('ref_axis',(0.532032076515336,0.846724199228284,0.)) ;
#34566=DIRECTION('center_axis',(-0.707106781186547,0.707106781186548,0.)) ;
#34567=DIRECTION('ref_axis',(0.707106781186548,0.707106781186547,0.)) ;
#34568=DIRECTION('center_axis',(0.,0.,1.)) ;
#34569=DIRECTION('ref_axis',(1.,0.,0.)) ;
#34570=DIRECTION('center_axis',(0.707106781186547,-0.707106781186548,0.)) ;
#34571=DIRECTION('ref_axis',(0.707106781186548,0.707106781186547,0.)) ;
#34572=DIRECTION('center_axis',(-0.532032076515336,0.846724199228284,0.)) ;
#34573=DIRECTION('ref_axis',(0.846724199228284,0.532032076515336,0.)) ;
#34574=DIRECTION('center_axis',(0.,0.,1.)) ;
#34575=DIRECTION('ref_axis',(1.,0.,0.)) ;
#34576=DIRECTION('center_axis',(0.532032076515336,-0.846724199228284,0.)) ;
#34577=DIRECTION('ref_axis',(0.846724199228284,0.532032076515336,0.)) ;
#34578=DIRECTION('center_axis',(-0.330279061955168,0.943883330308367,0.)) ;
#34579=DIRECTION('ref_axis',(0.943883330308367,0.330279061955168,0.)) ;
#34580=DIRECTION('center_axis',(0.,0.,1.)) ;
#34581=DIRECTION('ref_axis',(1.,0.,0.)) ;
#34582=DIRECTION('center_axis',(0.330279061955168,-0.943883330308367,0.)) ;
#34583=DIRECTION('ref_axis',(0.943883330308367,0.330279061955168,0.)) ;
#34584=DIRECTION('center_axis',(-0.111964476103307,0.993712209893243,0.)) ;
#34585=DIRECTION('ref_axis',(0.993712209893243,0.111964476103307,0.)) ;
#34586=DIRECTION('center_axis',(0.111964476103308,0.993712209893243,0.)) ;
#34587=DIRECTION('ref_axis',(0.993712209893243,-0.111964476103308,0.)) ;
#34588=DIRECTION('center_axis',(1.39008514084603E-14,1.,0.)) ;
#34589=DIRECTION('ref_axis',(1.,-1.39008514084603E-14,0.)) ;
#34590=DIRECTION('center_axis',(1.39008514084603E-14,1.,0.)) ;
#34591=DIRECTION('ref_axis',(1.,-1.39008514084603E-14,0.)) ;
#34592=DIRECTION('',(-0.111964476103308,-0.993712209893243,0.)) ;
#34593=DIRECTION('center_axis',(-0.222520933956317,-0.974927912181823,0.)) ;
#34594=DIRECTION('ref_axis',(0.974927912181823,-0.222520933956317,0.)) ;
#34595=DIRECTION('center_axis',(-0.222520933956317,-0.974927912181823,0.)) ;
#34596=DIRECTION('ref_axis',(0.974927912181823,-0.222520933956317,0.)) ;
#34597=DIRECTION('center_axis',(0.330279061955167,0.943883330308368,0.)) ;
#34598=DIRECTION('ref_axis',(0.943883330308368,-0.330279061955167,0.)) ;
#34599=DIRECTION('',(-0.330279061955167,-0.943883330308368,0.)) ;
#34600=DIRECTION('center_axis',(-0.433883739117561,-0.900968867902418,0.)) ;
#34601=DIRECTION('ref_axis',(0.900968867902418,-0.433883739117561,0.)) ;
#34602=DIRECTION('center_axis',(-0.433883739117561,-0.900968867902418,0.)) ;
#34603=DIRECTION('ref_axis',(0.900968867902418,-0.433883739117561,0.)) ;
#34604=DIRECTION('center_axis',(0.532032076515336,0.846724199228284,0.)) ;
#34605=DIRECTION('ref_axis',(0.846724199228285,-0.532032076515336,0.)) ;
#34606=DIRECTION('',(-0.532032076515336,-0.846724199228284,0.)) ;
#34607=DIRECTION('center_axis',(-0.623489801858739,-0.781831482468025,0.)) ;
#34608=DIRECTION('ref_axis',(0.781831482468025,-0.623489801858739,0.)) ;
#34609=DIRECTION('center_axis',(-0.623489801858739,-0.781831482468025,0.)) ;
#34610=DIRECTION('ref_axis',(0.781831482468025,-0.623489801858739,0.)) ;
#34611=DIRECTION('center_axis',(0.707106781186548,0.707106781186547,0.)) ;
#34612=DIRECTION('ref_axis',(0.707106781186547,-0.707106781186548,0.)) ;
#34613=DIRECTION('',(-0.707106781186548,-0.707106781186547,0.)) ;
#34614=DIRECTION('center_axis',(-0.781831482468025,-0.623489801858739,0.)) ;
#34615=DIRECTION('ref_axis',(0.623489801858739,-0.781831482468025,0.)) ;
#34616=DIRECTION('center_axis',(-0.781831482468025,-0.623489801858739,0.)) ;
#34617=DIRECTION('ref_axis',(0.623489801858739,-0.781831482468025,0.)) ;
#34618=DIRECTION('center_axis',(0.846724199228284,0.532032076515337,0.)) ;
#34619=DIRECTION('ref_axis',(0.532032076515337,-0.846724199228284,0.)) ;
#34620=DIRECTION('',(-0.846724199228284,-0.532032076515337,0.)) ;
#34621=DIRECTION('center_axis',(-0.900968867902421,-0.433883739117553,0.)) ;
#34622=DIRECTION('ref_axis',(0.433883739117553,-0.900968867902422,0.)) ;
#34623=DIRECTION('center_axis',(-0.900968867902421,-0.433883739117553,0.)) ;
#34624=DIRECTION('ref_axis',(0.433883739117553,-0.900968867902422,0.)) ;
#34625=DIRECTION('center_axis',(0.943883330308368,0.330279061955166,0.)) ;
#34626=DIRECTION('ref_axis',(0.330279061955166,-0.943883330308368,0.)) ;
#34627=DIRECTION('',(-0.943883330308368,-0.330279061955166,0.)) ;
#34628=DIRECTION('center_axis',(-0.974927912181825,-0.222520933956307,0.)) ;
#34629=DIRECTION('ref_axis',(0.222520933956307,-0.974927912181825,0.)) ;
#34630=DIRECTION('center_axis',(-0.974927912181825,-0.222520933956307,0.)) ;
#34631=DIRECTION('ref_axis',(0.222520933956307,-0.974927912181825,0.)) ;
#34632=DIRECTION('center_axis',(0.993712209893243,0.111964476103307,0.)) ;
#34633=DIRECTION('ref_axis',(0.111964476103307,-0.993712209893243,0.)) ;
#34634=DIRECTION('',(-0.993712209893243,-0.111964476103307,0.)) ;
#34635=DIRECTION('center_axis',(-1.,1.19150154929659E-14,0.)) ;
#34636=DIRECTION('ref_axis',(-1.19150154929659E-14,-1.,0.)) ;
#34637=DIRECTION('center_axis',(-1.,1.19150154929659E-14,0.)) ;
#34638=DIRECTION('ref_axis',(-1.19150154929659E-14,-1.,0.)) ;
#34639=DIRECTION('center_axis',(0.993712209893243,-0.111964476103307,0.)) ;
#34640=DIRECTION('ref_axis',(0.111964476103307,0.993712209893243,0.)) ;
#34641=DIRECTION('',(-0.993712209893243,0.111964476103307,0.)) ;
#34642=DIRECTION('center_axis',(-0.974927912181822,0.22252093395632,0.)) ;
#34643=DIRECTION('ref_axis',(0.22252093395632,0.974927912181822,0.)) ;
#34644=DIRECTION('center_axis',(0.943883330308367,-0.330279061955168,0.)) ;
#34645=DIRECTION('ref_axis',(0.330279061955168,0.943883330308367,0.)) ;
#34646=DIRECTION('',(-0.943883330308367,0.330279061955168,0.)) ;
#34647=DIRECTION('center_axis',(-0.900968867902414,0.433883739117568,0.)) ;
#34648=DIRECTION('ref_axis',(0.433883739117568,0.900968867902414,0.)) ;
#34649=DIRECTION('center_axis',(0.846724199228284,-0.532032076515337,0.)) ;
#34650=DIRECTION('ref_axis',(0.532032076515337,0.846724199228284,0.)) ;
#34651=DIRECTION('',(-0.846724199228284,0.532032076515337,0.)) ;
#34652=DIRECTION('center_axis',(-0.781831482468023,0.623489801858742,0.)) ;
#34653=DIRECTION('ref_axis',(0.623489801858742,0.781831482468023,0.)) ;
#34654=DIRECTION('center_axis',(0.707106781186548,-0.707106781186547,0.)) ;
#34655=DIRECTION('ref_axis',(0.707106781186547,0.707106781186548,0.)) ;
#34656=DIRECTION('',(-0.707106781186548,0.707106781186547,0.)) ;
#34657=DIRECTION('center_axis',(-0.62348980185874,0.781831482468024,0.)) ;
#34658=DIRECTION('ref_axis',(0.781831482468024,0.62348980185874,0.)) ;
#34659=DIRECTION('center_axis',(0.532032076515336,-0.846724199228284,0.)) ;
#34660=DIRECTION('ref_axis',(0.846724199228284,0.532032076515336,0.)) ;
#34661=DIRECTION('',(-0.532032076515336,0.846724199228284,0.)) ;
#34662=DIRECTION('center_axis',(-0.433883739117548,0.900968867902424,0.)) ;
#34663=DIRECTION('ref_axis',(0.900968867902424,0.433883739117548,0.)) ;
#34664=DIRECTION('center_axis',(0.330279061955167,-0.943883330308368,0.)) ;
#34665=DIRECTION('ref_axis',(0.943883330308368,0.330279061955167,0.)) ;
#34666=DIRECTION('',(-0.330279061955167,0.943883330308368,0.)) ;
#34667=DIRECTION('center_axis',(-0.222520933956297,0.974927912181828,0.)) ;
#34668=DIRECTION('ref_axis',(0.974927912181828,0.222520933956297,0.)) ;
#34669=DIRECTION('center_axis',(0.111964476103307,-0.993712209893243,0.)) ;
#34670=DIRECTION('ref_axis',(0.993712209893243,0.111964476103307,0.)) ;
#34671=DIRECTION('',(-0.111964476103307,0.993712209893243,0.)) ;
#34672=DIRECTION('center_axis',(1.14737186228561E-14,1.,0.)) ;
#34673=DIRECTION('ref_axis',(1.,-1.1487509150047E-14,0.)) ;
#34674=DIRECTION('center_axis',(-0.111964476103307,-0.993712209893243,0.)) ;
#34675=DIRECTION('ref_axis',(0.993712209893243,-0.111964476103307,0.)) ;
#34676=DIRECTION('',(0.111964476103307,0.993712209893243,0.)) ;
#34677=DIRECTION('center_axis',(0.22252093395631,0.974927912181825,0.)) ;
#34678=DIRECTION('ref_axis',(0.974927912181825,-0.22252093395631,0.)) ;
#34679=DIRECTION('center_axis',(-0.330279061955167,-0.943883330308367,0.)) ;
#34680=DIRECTION('ref_axis',(0.943883330308368,-0.330279061955167,0.)) ;
#34681=DIRECTION('',(0.330279061955167,0.943883330308367,0.)) ;
#34682=DIRECTION('center_axis',(0.433883739117568,0.900968867902414,0.)) ;
#34683=DIRECTION('ref_axis',(0.900968867902414,-0.433883739117568,0.)) ;
#34684=DIRECTION('center_axis',(-0.532032076515337,-0.846724199228284,0.)) ;
#34685=DIRECTION('ref_axis',(0.846724199228284,-0.532032076515337,0.)) ;
#34686=DIRECTION('',(0.532032076515337,0.846724199228284,0.)) ;
#34687=DIRECTION('center_axis',(0.623489801858745,0.78183148246802,0.)) ;
#34688=DIRECTION('ref_axis',(0.78183148246802,-0.623489801858745,0.)) ;
#34689=DIRECTION('center_axis',(-0.707106781186548,-0.707106781186548,0.)) ;
#34690=DIRECTION('ref_axis',(0.707106781186548,-0.707106781186548,0.)) ;
#34691=DIRECTION('',(0.707106781186548,0.707106781186548,0.)) ;
#34692=DIRECTION('center_axis',(0.781831482468033,0.623489801858729,0.)) ;
#34693=DIRECTION('ref_axis',(0.623489801858729,-0.781831482468033,0.)) ;
#34694=DIRECTION('center_axis',(-0.846724199228285,-0.532032076515336,0.)) ;
#34695=DIRECTION('ref_axis',(0.532032076515336,-0.846724199228285,0.)) ;
#34696=DIRECTION('',(0.846724199228285,0.532032076515336,0.)) ;
#34697=DIRECTION('center_axis',(0.900968867902424,0.433883739117548,0.)) ;
#34698=DIRECTION('ref_axis',(0.433883739117548,-0.900968867902424,0.)) ;
#34699=DIRECTION('center_axis',(-0.943883330308367,-0.330279061955168,0.)) ;
#34700=DIRECTION('ref_axis',(0.330279061955168,-0.943883330308367,0.)) ;
#34701=DIRECTION('',(0.943883330308367,0.330279061955168,0.)) ;
#34702=DIRECTION('center_axis',(0.974927912181826,0.222520933956302,0.)) ;
#34703=DIRECTION('ref_axis',(0.222520933956302,-0.974927912181826,0.)) ;
#34704=DIRECTION('center_axis',(-0.993712209893243,-0.111964476103307,0.)) ;
#34705=DIRECTION('ref_axis',(0.111964476103307,-0.993712209893243,0.)) ;
#34706=DIRECTION('',(0.993712209893243,0.111964476103307,0.)) ;
#34707=DIRECTION('center_axis',(1.,-1.34595545383504E-14,0.)) ;
#34708=DIRECTION('ref_axis',(-1.34733450655413E-14,-1.,0.)) ;
#34709=DIRECTION('center_axis',(1.,-1.34595545383504E-14,0.)) ;
#34710=DIRECTION('ref_axis',(-1.34733450655413E-14,-1.,0.)) ;
#34711=DIRECTION('center_axis',(-0.993712209893243,0.111964476103307,0.)) ;
#34712=DIRECTION('ref_axis',(0.111964476103307,0.993712209893243,0.)) ;
#34713=DIRECTION('',(0.993712209893243,-0.111964476103307,0.)) ;
#34714=DIRECTION('center_axis',(0.974927912181822,-0.222520933956322,0.)) ;
#34715=DIRECTION('ref_axis',(0.222520933956322,0.974927912181822,0.)) ;
#34716=DIRECTION('center_axis',(0.974927912181822,-0.222520933956322,0.)) ;
#34717=DIRECTION('ref_axis',(0.222520933956322,0.974927912181822,0.)) ;
#34718=DIRECTION('center_axis',(-0.943883330308367,0.330279061955168,0.)) ;
#34719=DIRECTION('ref_axis',(0.330279061955168,0.943883330308367,0.)) ;
#34720=DIRECTION('',(0.943883330308367,-0.330279061955168,0.)) ;
#34721=DIRECTION('center_axis',(0.900968867902422,-0.433883739117553,0.)) ;
#34722=DIRECTION('ref_axis',(0.433883739117553,0.900968867902422,0.)) ;
#34723=DIRECTION('center_axis',(0.900968867902422,-0.433883739117553,0.)) ;
#34724=DIRECTION('ref_axis',(0.433883739117553,0.900968867902422,0.)) ;
#34725=DIRECTION('center_axis',(-0.846724199228284,0.532032076515336,0.)) ;
#34726=DIRECTION('ref_axis',(0.532032076515336,0.846724199228284,0.)) ;
#34727=DIRECTION('',(0.846724199228284,-0.532032076515336,0.)) ;
#34728=DIRECTION('center_axis',(0.781831482468019,-0.623489801858747,0.)) ;
#34729=DIRECTION('ref_axis',(0.623489801858747,0.781831482468019,0.)) ;
#34730=DIRECTION('center_axis',(0.781831482468019,-0.623489801858747,0.)) ;
#34731=DIRECTION('ref_axis',(0.623489801858747,0.781831482468019,0.)) ;
#34732=DIRECTION('center_axis',(-0.707106781186547,0.707106781186548,0.)) ;
#34733=DIRECTION('ref_axis',(0.707106781186548,0.707106781186547,0.)) ;
#34734=DIRECTION('',(0.707106781186547,-0.707106781186548,0.)) ;
#34735=DIRECTION('center_axis',(0.623489801858735,-0.781831482468028,0.)) ;
#34736=DIRECTION('ref_axis',(0.781831482468028,0.623489801858735,0.)) ;
#34737=DIRECTION('center_axis',(0.623489801858735,-0.781831482468028,0.)) ;
#34738=DIRECTION('ref_axis',(0.781831482468028,0.623489801858735,0.)) ;
#34739=DIRECTION('center_axis',(-0.532032076515336,0.846724199228284,0.)) ;
#34740=DIRECTION('ref_axis',(0.846724199228284,0.532032076515336,0.)) ;
#34741=DIRECTION('',(0.532032076515336,-0.846724199228284,0.)) ;
#34742=DIRECTION('center_axis',(0.433883739117553,-0.900968867902422,0.)) ;
#34743=DIRECTION('ref_axis',(0.900968867902422,0.433883739117553,0.)) ;
#34744=DIRECTION('center_axis',(0.433883739117553,-0.900968867902422,0.)) ;
#34745=DIRECTION('ref_axis',(0.900968867902422,0.433883739117553,0.)) ;
#34746=DIRECTION('center_axis',(-0.330279061955168,0.943883330308367,0.)) ;
#34747=DIRECTION('ref_axis',(0.943883330308367,0.330279061955168,0.)) ;
#34748=DIRECTION('',(0.330279061955168,-0.943883330308367,0.)) ;
#34749=DIRECTION('center_axis',(0.222520933956303,-0.974927912181826,0.)) ;
#34750=DIRECTION('ref_axis',(0.974927912181826,0.222520933956303,0.)) ;
#34751=DIRECTION('center_axis',(0.222520933956303,-0.974927912181826,0.)) ;
#34752=DIRECTION('ref_axis',(0.974927912181826,0.222520933956303,0.)) ;
#34753=DIRECTION('center_axis',(-0.111964476103307,0.993712209893243,0.)) ;
#34754=DIRECTION('ref_axis',(0.993712209893243,0.111964476103307,0.)) ;
#34755=DIRECTION('',(0.111964476103307,-0.993712209893243,0.)) ;
#43441=CARTESIAN_POINT('',(0.,0.,0.)) ;
#43442=CARTESIAN_POINT('Origin',(31.,0.,70.)) ;
#43443=CARTESIAN_POINT('',(30.9999999999999,-2.15655990727168E-15,72.)) ;
#43444=CARTESIAN_POINT('',(30.9999999999999,-2.15655990727168E-15,68.)) ;
#43445=CARTESIAN_POINT('Origin',(31.,-7.99360577730113E-15,70.)) ;
#43446=CARTESIAN_POINT('Origin',(31.,0.,70.)) ;
#43447=CARTESIAN_POINT('Origin',(30.2227652776365,-6.89814895264575,70.)) ;
#43448=CARTESIAN_POINT('',(30.2227652776365,-6.89814895264575,68.)) ;
#43449=CARTESIAN_POINT('',(30.2227652776365,-6.89814895264575,72.)) ;
#43450=CARTESIAN_POINT('Origin',(30.2227652776365,-6.89814895264575,70.)) ;
#43451=CARTESIAN_POINT('Origin',(30.2227652776365,-6.89814895264576,70.)) ;
#43452=CARTESIAN_POINT('Origin',(27.930034904975,-13.4503959126443,70.)) ;
#43453=CARTESIAN_POINT('',(27.930034904975,-13.4503959126443,68.)) ;
#43454=CARTESIAN_POINT('',(27.930034904975,-13.4503959126443,72.)) ;
#43455=CARTESIAN_POINT('Origin',(27.930034904975,-13.4503959126443,70.)) ;
#43456=CARTESIAN_POINT('Origin',(27.930034904975,-13.4503959126443,70.)) ;
#43457=CARTESIAN_POINT('Origin',(24.2367759565089,-19.3281838576207,70.)) ;
#43458=CARTESIAN_POINT('',(24.2367759565089,-19.3281838576207,68.)) ;
#43459=CARTESIAN_POINT('',(24.2367759565089,-19.3281838576207,72.)) ;
#43460=CARTESIAN_POINT('Origin',(24.2367759565089,-19.3281838576207,70.)) ;
#43461=CARTESIAN_POINT('Origin',(24.2367759565089,-19.3281838576208,70.)) ;
#43462=CARTESIAN_POINT('Origin',(19.3281838576207,-24.2367759565089,70.)) ;
#43463=CARTESIAN_POINT('',(19.3281838576208,-24.236775956509,68.)) ;
#43464=CARTESIAN_POINT('',(19.3281838576208,-24.236775956509,72.)) ;
#43465=CARTESIAN_POINT('Origin',(19.3281838576207,-24.2367759565089,70.)) ;
#43466=CARTESIAN_POINT('Origin',(19.3281838576207,-24.2367759565089,70.)) ;
#43467=CARTESIAN_POINT('Origin',(13.4503959126443,-27.930034904975,70.)) ;
#43468=CARTESIAN_POINT('',(13.4503959126442,-27.9300349049749,68.)) ;
#43469=CARTESIAN_POINT('',(13.4503959126442,-27.9300349049749,72.)) ;
#43470=CARTESIAN_POINT('Origin',(13.4503959126443,-27.930034904975,70.)) ;
#43471=CARTESIAN_POINT('Origin',(13.4503959126443,-27.930034904975,70.)) ;
#43472=CARTESIAN_POINT('Origin',(6.89814895264571,-30.2227652776365,70.)) ;
#43473=CARTESIAN_POINT('',(6.89814895264574,-30.2227652776366,68.)) ;
#43474=CARTESIAN_POINT('',(6.89814895264574,-30.2227652776366,72.)) ;
#43475=CARTESIAN_POINT('Origin',(6.89814895264571,-30.2227652776365,70.)) ;
#43476=CARTESIAN_POINT('Origin',(6.89814895264571,-30.2227652776365,70.)) ;
#43477=CARTESIAN_POINT('Origin',(-5.69460761603519E-15,-31.,70.)) ;
#43478=CARTESIAN_POINT('',(-9.22043443155371E-15,-31.,68.)) ;
#43479=CARTESIAN_POINT('',(-9.22043443155371E-15,-31.,72.)) ;
#43480=CARTESIAN_POINT('Origin',(-5.32907051820075E-15,-31.,70.)) ;
#43481=CARTESIAN_POINT('',(-0.223928952206608,-32.9874244197865,70.)) ;
#43482=CARTESIAN_POINT('Origin',(-5.32907051820075E-15,-31.,70.)) ;
#43483=CARTESIAN_POINT('Origin',(-5.32907051820075E-15,-31.,70.)) ;
#43484=CARTESIAN_POINT('Origin',(-6.89814895264575,-30.2227652776365,70.)) ;
#43485=CARTESIAN_POINT('',(-6.89814895264576,-30.2227652776366,68.)) ;
#43486=CARTESIAN_POINT('',(-7.12207790485237,-32.210189697423,70.)) ;
#43487=CARTESIAN_POINT('Origin',(-6.89814895264575,-30.2227652776365,70.)) ;
#43488=CARTESIAN_POINT('',(-6.89814895264576,-30.2227652776366,72.)) ;
#43489=CARTESIAN_POINT('Origin',(-6.89814895264575,-30.2227652776365,70.)) ;
#43490=CARTESIAN_POINT('',(-7.55870707655606,-32.1105319382533,70.)) ;
#43491=CARTESIAN_POINT('Origin',(-6.89814895264575,-30.2227652776365,70.)) ;
#43492=CARTESIAN_POINT('Origin',(-6.89814895264575,-30.2227652776365,70.)) ;
#43493=CARTESIAN_POINT('Origin',(-13.4503959126443,-27.930034904975,70.)) ;
#43494=CARTESIAN_POINT('',(-13.4503959126443,-27.930034904975,68.)) ;
#43495=CARTESIAN_POINT('',(-14.1109540365546,-29.8178015655917,70.)) ;
#43496=CARTESIAN_POINT('Origin',(-13.4503959126443,-27.930034904975,70.)) ;
#43497=CARTESIAN_POINT('',(-13.4503959126443,-27.930034904975,72.)) ;
#43498=CARTESIAN_POINT('Origin',(-13.4503959126443,-27.930034904975,70.)) ;
#43499=CARTESIAN_POINT('',(-14.514460065675,-29.6234833034316,70.)) ;
#43500=CARTESIAN_POINT('Origin',(-13.4503959126443,-27.930034904975,70.)) ;
#43501=CARTESIAN_POINT('Origin',(-13.4503959126443,-27.930034904975,70.)) ;
#43502=CARTESIAN_POINT('Origin',(-19.3281838576207,-24.2367759565089,70.)) ;
#43503=CARTESIAN_POINT('',(-19.3281838576207,-24.2367759565089,68.)) ;
#43504=CARTESIAN_POINT('',(-20.3922480106514,-25.9302243549655,70.)) ;
#43505=CARTESIAN_POINT('Origin',(-19.3281838576207,-24.2367759565089,70.)) ;
#43506=CARTESIAN_POINT('',(-19.3281838576207,-24.2367759565089,72.)) ;
#43507=CARTESIAN_POINT('Origin',(-19.3281838576207,-24.2367759565089,70.)) ;
#43508=CARTESIAN_POINT('',(-20.7423974199938,-25.650989518882,70.)) ;
#43509=CARTESIAN_POINT('Origin',(-19.3281838576207,-24.2367759565089,70.)) ;
#43510=CARTESIAN_POINT('Origin',(-19.3281838576207,-24.2367759565089,70.)) ;
#43511=CARTESIAN_POINT('Origin',(-24.2367759565089,-19.3281838576208,70.)) ;
#43512=CARTESIAN_POINT('',(-24.236775956509,-19.3281838576208,68.)) ;
#43513=CARTESIAN_POINT('',(-25.650989518882,-20.7423974199938,70.)) ;
#43514=CARTESIAN_POINT('Origin',(-24.2367759565089,-19.3281838576208,70.)) ;
#43515=CARTESIAN_POINT('',(-24.236775956509,-19.3281838576208,72.)) ;
#43516=CARTESIAN_POINT('Origin',(-24.2367759565089,-19.3281838576208,70.)) ;
#43517=CARTESIAN_POINT('',(-25.9302243549655,-20.3922480106514,70.)) ;
#43518=CARTESIAN_POINT('Origin',(-24.2367759565089,-19.3281838576208,70.)) ;
#43519=CARTESIAN_POINT('Origin',(-24.2367759565089,-19.3281838576208,70.)) ;
#43520=CARTESIAN_POINT('Origin',(-27.930034904975,-13.4503959126443,70.)) ;
#43521=CARTESIAN_POINT('',(-27.930034904975,-13.4503959126443,68.)) ;
#43522=CARTESIAN_POINT('',(-29.6234833034316,-14.514460065675,70.)) ;
#43523=CARTESIAN_POINT('Origin',(-27.930034904975,-13.4503959126443,70.)) ;
#43524=CARTESIAN_POINT('',(-27.930034904975,-13.4503959126443,72.)) ;
#43525=CARTESIAN_POINT('Origin',(-27.930034904975,-13.4503959126443,70.)) ;
#43526=CARTESIAN_POINT('',(-29.8178015655917,-14.1109540365547,70.)) ;
#43527=CARTESIAN_POINT('Origin',(-27.930034904975,-13.4503959126443,70.)) ;
#43528=CARTESIAN_POINT('Origin',(-27.930034904975,-13.4503959126443,70.)) ;
#43529=CARTESIAN_POINT('Origin',(-30.2227652776365,-6.89814895264573,70.)) ;
#43530=CARTESIAN_POINT('',(-30.2227652776365,-6.89814895264572,68.)) ;
#43531=CARTESIAN_POINT('',(-32.1105319382533,-7.55870707655606,70.)) ;
#43532=CARTESIAN_POINT('Origin',(-30.2227652776365,-6.89814895264573,70.)) ;
#43533=CARTESIAN_POINT('',(-30.2227652776365,-6.89814895264572,72.)) ;
#43534=CARTESIAN_POINT('Origin',(-30.2227652776365,-6.89814895264573,70.)) ;
#43535=CARTESIAN_POINT('',(-32.210189697423,-7.12207790485236,70.)) ;
#43536=CARTESIAN_POINT('Origin',(-30.2227652776365,-6.89814895264573,70.)) ;
#43537=CARTESIAN_POINT('Origin',(-30.2227652776365,-6.89814895264573,70.)) ;
#43538=CARTESIAN_POINT('Origin',(-31.,3.7964050773568E-15,70.)) ;
#43539=CARTESIAN_POINT('',(-31.,7.44407759215346E-15,68.)) ;
#43540=CARTESIAN_POINT('',(-32.9874244197865,-0.223928952206611,70.)) ;
#43541=CARTESIAN_POINT('Origin',(-31.,3.5527136788005E-15,70.)) ;
#43542=CARTESIAN_POINT('',(-31.,7.44407759215346E-15,72.)) ;
#43543=CARTESIAN_POINT('Origin',(-31.,3.5527136788005E-15,70.)) ;
#43544=CARTESIAN_POINT('',(-32.9874244197865,0.2239289522066,70.)) ;
#43545=CARTESIAN_POINT('Origin',(-31.,3.5527136788005E-15,70.)) ;
#43546=CARTESIAN_POINT('Origin',(-31.,3.5527136788005E-15,70.)) ;
#43547=CARTESIAN_POINT('Origin',(-30.2227652776365,6.89814895264574,70.)) ;
#43548=CARTESIAN_POINT('',(-30.2227652776366,6.89814895264574,68.)) ;
#43549=CARTESIAN_POINT('',(-32.210189697423,7.12207790485236,70.)) ;
#43550=CARTESIAN_POINT('Origin',(-30.2227652776365,6.89814895264574,70.)) ;
#43551=CARTESIAN_POINT('',(-30.2227652776366,6.89814895264574,72.)) ;
#43552=CARTESIAN_POINT('Origin',(-30.2227652776365,6.89814895264574,70.)) ;
#43553=CARTESIAN_POINT('',(-32.1105319382533,7.55870707655606,70.)) ;
#43554=CARTESIAN_POINT('Origin',(-30.2227652776365,6.89814895264574,70.)) ;
#43555=CARTESIAN_POINT('Origin',(-30.2227652776365,6.89814895264574,70.)) ;
#43556=CARTESIAN_POINT('Origin',(-27.930034904975,13.4503959126443,70.)) ;
#43557=CARTESIAN_POINT('',(-27.930034904975,13.4503959126443,68.)) ;
#43558=CARTESIAN_POINT('',(-29.8178015655917,14.1109540365546,70.)) ;
#43559=CARTESIAN_POINT('Origin',(-27.930034904975,13.4503959126443,70.)) ;
#43560=CARTESIAN_POINT('',(-27.930034904975,13.4503959126443,72.)) ;
#43561=CARTESIAN_POINT('Origin',(-27.930034904975,13.4503959126443,70.)) ;
#43562=CARTESIAN_POINT('',(-29.6234833034316,14.514460065675,70.)) ;
#43563=CARTESIAN_POINT('Origin',(-27.930034904975,13.4503959126443,70.)) ;
#43564=CARTESIAN_POINT('Origin',(-27.930034904975,13.4503959126443,70.)) ;
#43565=CARTESIAN_POINT('Origin',(-24.2367759565089,19.3281838576208,70.)) ;
#43566=CARTESIAN_POINT('',(-24.236775956509,19.3281838576208,68.)) ;
#43567=CARTESIAN_POINT('',(-25.9302243549655,20.3922480106514,70.)) ;
#43568=CARTESIAN_POINT('Origin',(-24.2367759565089,19.3281838576208,70.)) ;
#43569=CARTESIAN_POINT('',(-24.236775956509,19.3281838576208,72.)) ;
#43570=CARTESIAN_POINT('Origin',(-24.2367759565089,19.3281838576208,70.)) ;
#43571=CARTESIAN_POINT('',(-25.650989518882,20.7423974199938,70.)) ;
#43572=CARTESIAN_POINT('Origin',(-24.2367759565089,19.3281838576208,70.)) ;
#43573=CARTESIAN_POINT('Origin',(-24.2367759565089,19.3281838576208,70.)) ;
#43574=CARTESIAN_POINT('Origin',(-19.3281838576207,24.2367759565089,70.)) ;
#43575=CARTESIAN_POINT('',(-19.3281838576207,24.2367759565089,68.)) ;
#43576=CARTESIAN_POINT('',(-20.7423974199938,25.650989518882,70.)) ;
#43577=CARTESIAN_POINT('Origin',(-19.3281838576207,24.2367759565089,70.)) ;
#43578=CARTESIAN_POINT('',(-19.3281838576207,24.2367759565089,72.)) ;
#43579=CARTESIAN_POINT('Origin',(-19.3281838576207,24.2367759565089,70.)) ;
#43580=CARTESIAN_POINT('',(-20.3922480106514,25.9302243549655,70.)) ;
#43581=CARTESIAN_POINT('Origin',(-19.3281838576207,24.2367759565089,70.)) ;
#43582=CARTESIAN_POINT('Origin',(-19.3281838576207,24.2367759565089,70.)) ;
#43583=CARTESIAN_POINT('Origin',(-13.4503959126443,27.930034904975,70.)) ;
#43584=CARTESIAN_POINT('',(-13.4503959126443,27.930034904975,68.)) ;
#43585=CARTESIAN_POINT('',(-14.514460065675,29.6234833034316,70.)) ;
#43586=CARTESIAN_POINT('Origin',(-13.4503959126443,27.930034904975,70.)) ;
#43587=CARTESIAN_POINT('',(-13.4503959126443,27.930034904975,72.)) ;
#43588=CARTESIAN_POINT('Origin',(-13.4503959126443,27.930034904975,70.)) ;
#43589=CARTESIAN_POINT('',(-14.1109540365547,29.8178015655917,70.)) ;
#43590=CARTESIAN_POINT('Origin',(-13.4503959126443,27.930034904975,70.)) ;
#43591=CARTESIAN_POINT('Origin',(-13.4503959126443,27.930034904975,70.)) ;
#43592=CARTESIAN_POINT('Origin',(-6.89814895264574,30.2227652776365,70.)) ;
#43593=CARTESIAN_POINT('',(-6.89814895264573,30.2227652776365,68.)) ;
#43594=CARTESIAN_POINT('',(-7.55870707655608,32.1105319382533,70.)) ;
#43595=CARTESIAN_POINT('Origin',(-6.89814895264574,30.2227652776365,70.)) ;
#43596=CARTESIAN_POINT('',(-6.89814895264573,30.2227652776365,72.)) ;
#43597=CARTESIAN_POINT('Origin',(-6.89814895264574,30.2227652776365,70.)) ;
#43598=CARTESIAN_POINT('',(-7.12207790485237,32.210189697423,70.)) ;
#43599=CARTESIAN_POINT('Origin',(-6.89814895264574,30.2227652776365,70.)) ;
#43600=CARTESIAN_POINT('Origin',(-6.89814895264574,30.2227652776365,70.)) ;
#43601=CARTESIAN_POINT('Origin',(1.8982025386784E-15,31.,70.)) ;
#43602=CARTESIAN_POINT('',(5.66772075275322E-15,31.,68.)) ;
#43603=CARTESIAN_POINT('',(-0.223928952206612,32.9874244197865,70.)) ;
#43604=CARTESIAN_POINT('Origin',(1.77635683940025E-15,31.,70.)) ;
#43605=CARTESIAN_POINT('',(5.66772075275322E-15,31.,72.)) ;
#43606=CARTESIAN_POINT('Origin',(1.77635683940025E-15,31.,70.)) ;
#43607=CARTESIAN_POINT('Origin',(1.77635683940025E-15,31.,70.)) ;
#43608=CARTESIAN_POINT('Origin',(6.89814895264575,30.2227652776365,70.)) ;
#43609=CARTESIAN_POINT('',(6.89814895264576,30.2227652776366,68.)) ;
#43610=CARTESIAN_POINT('',(6.89814895264576,30.2227652776366,72.)) ;
#43611=CARTESIAN_POINT('Origin',(6.89814895264575,30.2227652776365,70.)) ;
#43612=CARTESIAN_POINT('Origin',(6.89814895264575,30.2227652776365,70.)) ;
#43613=CARTESIAN_POINT('Origin',(13.4503959126443,27.930034904975,70.)) ;
#43614=CARTESIAN_POINT('',(13.4503959126443,27.930034904975,68.)) ;
#43615=CARTESIAN_POINT('',(13.4503959126443,27.930034904975,72.)) ;
#43616=CARTESIAN_POINT('Origin',(13.4503959126443,27.930034904975,70.)) ;
#43617=CARTESIAN_POINT('Origin',(13.4503959126443,27.930034904975,70.)) ;
#43618=CARTESIAN_POINT('Origin',(19.3281838576207,24.2367759565089,70.)) ;
#43619=CARTESIAN_POINT('',(19.3281838576208,24.236775956509,68.)) ;
#43620=CARTESIAN_POINT('',(19.3281838576208,24.236775956509,72.)) ;
#43621=CARTESIAN_POINT('Origin',(19.3281838576207,24.2367759565089,70.)) ;
#43622=CARTESIAN_POINT('Origin',(19.3281838576207,24.2367759565089,70.)) ;
#43623=CARTESIAN_POINT('Origin',(24.2367759565089,19.3281838576207,70.)) ;
#43624=CARTESIAN_POINT('',(24.2367759565089,19.3281838576207,68.)) ;
#43625=CARTESIAN_POINT('',(24.2367759565089,19.3281838576207,72.)) ;
#43626=CARTESIAN_POINT('Origin',(24.2367759565089,19.3281838576207,70.)) ;
#43627=CARTESIAN_POINT('Origin',(24.2367759565089,19.3281838576207,70.)) ;
#43628=CARTESIAN_POINT('Origin',(27.930034904975,13.4503959126443,70.)) ;
#43629=CARTESIAN_POINT('',(27.930034904975,13.4503959126443,68.)) ;
#43630=CARTESIAN_POINT('',(27.930034904975,13.4503959126443,72.)) ;
#43631=CARTESIAN_POINT('Origin',(27.930034904975,13.4503959126443,70.)) ;
#43632=CARTESIAN_POINT('Origin',(27.930034904975,13.4503959126443,70.)) ;
#43633=CARTESIAN_POINT('Origin',(30.2227652776365,6.89814895264575,70.)) ;
#43634=CARTESIAN_POINT('',(30.2227652776365,6.89814895264574,68.)) ;
#43635=CARTESIAN_POINT('',(30.2227652776365,6.89814895264574,72.)) ;
#43636=CARTESIAN_POINT('Origin',(30.2227652776365,6.89814895264575,70.)) ;
#43637=CARTESIAN_POINT('Origin',(30.2227652776365,6.89814895264575,70.)) ;
#43638=CARTESIAN_POINT('Origin',(30.6113826388183,-3.44907447632288,70.)) ;
#43639=CARTESIAN_POINT('',(28.9873448468396,1.4210854715202E-14,70.)) ;
#43640=CARTESIAN_POINT('Origin',(31.,-1.37667655053519E-14,70.)) ;
#43641=CARTESIAN_POINT('Origin',(31.,-1.37667655053519E-14,70.)) ;
#43642=CARTESIAN_POINT('',(28.2605715912239,-6.4502910482325,70.)) ;
#43643=CARTESIAN_POINT('',(28.6239582190318,-3.22514552411626,70.)) ;
#43644=CARTESIAN_POINT('Origin',(30.2227652776365,-6.89814895264574,70.)) ;
#43645=CARTESIAN_POINT('Origin',(30.2227652776365,-6.89814895264574,70.)) ;
#43646=CARTESIAN_POINT('Origin',(29.0764000913058,-10.174272432645,70.)) ;
#43647=CARTESIAN_POINT('',(26.1166952701541,-12.5771375692368,70.)) ;
#43648=CARTESIAN_POINT('',(27.188633430689,-9.51371430873468,70.)) ;
#43649=CARTESIAN_POINT('Origin',(27.930034904975,-13.4503959126443,70.)) ;
#43650=CARTESIAN_POINT('Origin',(27.930034904975,-13.4503959126443,70.)) ;
#43651=CARTESIAN_POINT('Origin',(26.083405430742,-16.3892898851325,70.)) ;
#43652=CARTESIAN_POINT('',(22.6632187944166,-18.0733138949668,70.)) ;
#43653=CARTESIAN_POINT('',(24.3899570322854,-15.3252257321018,70.)) ;
#43654=CARTESIAN_POINT('Origin',(24.2367759565089,-19.3281838576207,70.)) ;
#43655=CARTESIAN_POINT('Origin',(24.2367759565089,-19.3281838576207,70.)) ;
#43656=CARTESIAN_POINT('Origin',(21.7824799070648,-21.7824799070648,70.)) ;
#43657=CARTESIAN_POINT('',(18.0733138949668,-22.6632187944167,70.)) ;
#43658=CARTESIAN_POINT('',(20.3682663446917,-20.3682663446917,70.)) ;
#43659=CARTESIAN_POINT('Origin',(19.3281838576207,-24.2367759565089,70.)) ;
#43660=CARTESIAN_POINT('Origin',(19.3281838576207,-24.2367759565089,70.)) ;
#43661=CARTESIAN_POINT('Origin',(16.3892898851325,-26.083405430742,70.)) ;
#43662=CARTESIAN_POINT('',(12.5771375692369,-26.1166952701541,70.)) ;
#43663=CARTESIAN_POINT('',(15.3252257321018,-24.3899570322854,70.)) ;
#43664=CARTESIAN_POINT('Origin',(13.4503959126443,-27.930034904975,70.)) ;
#43665=CARTESIAN_POINT('Origin',(13.4503959126443,-27.930034904975,70.)) ;
#43666=CARTESIAN_POINT('Origin',(10.174272432645,-29.0764000913058,70.)) ;
#43667=CARTESIAN_POINT('',(6.45029104823252,-28.2605715912239,70.)) ;
#43668=CARTESIAN_POINT('',(9.51371430873467,-27.188633430689,70.)) ;
#43669=CARTESIAN_POINT('Origin',(6.89814895264574,-30.2227652776365,70.)) ;
#43670=CARTESIAN_POINT('Origin',(6.89814895264574,-30.2227652776365,70.)) ;
#43671=CARTESIAN_POINT('Origin',(3.44907447632285,-30.6113826388183,70.)) ;
#43672=CARTESIAN_POINT('',(3.37507799486048E-14,-28.9873448468396,70.)) ;
#43673=CARTESIAN_POINT('',(3.22514552411624,-28.6239582190318,70.)) ;
#43674=CARTESIAN_POINT('Origin',(9.76996261670138E-15,-31.,70.)) ;
#43675=CARTESIAN_POINT('Origin',(9.76996261670138E-15,-31.,70.)) ;
#43676=CARTESIAN_POINT('Origin',(-3.44907447632288,-30.6113826388183,70.)) ;
#43677=CARTESIAN_POINT('',(-3.67300342852949,-32.5988070586048,70.)) ;
#43678=CARTESIAN_POINT('Origin',(-6.89814895264573,-30.2227652776365,70.)) ;
#43679=CARTESIAN_POINT('Origin',(-10.174272432645,-29.0764000913058,70.)) ;
#43680=CARTESIAN_POINT('',(-10.8348305565554,-30.9641667519225,70.)) ;
#43681=CARTESIAN_POINT('Origin',(-13.4503959126443,-27.930034904975,70.)) ;
#43682=CARTESIAN_POINT('Origin',(-16.3892898851325,-26.083405430742,70.)) ;
#43683=CARTESIAN_POINT('',(-17.4533540381632,-27.7768538291985,70.)) ;
#43684=CARTESIAN_POINT('Origin',(-19.3281838576207,-24.2367759565089,70.)) ;
#43685=CARTESIAN_POINT('Origin',(-21.7824799070648,-21.7824799070648,70.)) ;
#43686=CARTESIAN_POINT('',(-23.1966934694379,-23.1966934694379,70.)) ;
#43687=CARTESIAN_POINT('Origin',(-24.2367759565089,-19.3281838576207,70.)) ;
#43688=CARTESIAN_POINT('Origin',(-26.083405430742,-16.3892898851325,70.)) ;
#43689=CARTESIAN_POINT('',(-27.7768538291985,-17.4533540381632,70.)) ;
#43690=CARTESIAN_POINT('Origin',(-27.930034904975,-13.4503959126443,70.)) ;
#43691=CARTESIAN_POINT('Origin',(-29.0764000913058,-10.174272432645,70.)) ;
#43692=CARTESIAN_POINT('',(-30.9641667519225,-10.8348305565553,70.)) ;
#43693=CARTESIAN_POINT('Origin',(-30.2227652776365,-6.89814895264575,70.)) ;
#43694=CARTESIAN_POINT('Origin',(-30.6113826388183,-3.44907447632286,70.)) ;
#43695=CARTESIAN_POINT('',(-32.5988070586048,-3.67300342852948,70.)) ;
#43696=CARTESIAN_POINT('Origin',(-31.,-1.86517468137026E-14,70.)) ;
#43697=CARTESIAN_POINT('Origin',(-30.6113826388183,3.44907447632287,70.)) ;
#43698=CARTESIAN_POINT('',(-32.5988070586048,3.67300342852949,70.)) ;
#43699=CARTESIAN_POINT('Origin',(-30.2227652776365,6.89814895264573,70.)) ;
#43700=CARTESIAN_POINT('Origin',(-29.0764000913058,10.174272432645,70.)) ;
#43701=CARTESIAN_POINT('',(-30.9641667519225,10.8348305565554,70.)) ;
#43702=CARTESIAN_POINT('Origin',(-27.930034904975,13.4503959126443,70.)) ;
#43703=CARTESIAN_POINT('Origin',(-26.083405430742,16.3892898851325,70.)) ;
#43704=CARTESIAN_POINT('',(-27.7768538291985,17.4533540381632,70.)) ;
#43705=CARTESIAN_POINT('Origin',(-24.2367759565089,19.3281838576207,70.)) ;
#43706=CARTESIAN_POINT('Origin',(-21.7824799070648,21.7824799070648,70.)) ;
#43707=CARTESIAN_POINT('',(-23.1966934694379,23.1966934694379,70.)) ;
#43708=CARTESIAN_POINT('Origin',(-19.3281838576207,24.2367759565089,70.)) ;
#43709=CARTESIAN_POINT('Origin',(-16.3892898851325,26.083405430742,70.)) ;
#43710=CARTESIAN_POINT('',(-17.4533540381632,27.7768538291985,70.)) ;
#43711=CARTESIAN_POINT('Origin',(-13.4503959126443,27.930034904975,70.)) ;
#43712=CARTESIAN_POINT('Origin',(-10.174272432645,29.0764000913058,70.)) ;
#43713=CARTESIAN_POINT('',(-10.8348305565554,30.9641667519225,70.)) ;
#43714=CARTESIAN_POINT('Origin',(-6.89814895264576,30.2227652776365,70.)) ;
#43715=CARTESIAN_POINT('Origin',(-3.44907447632287,30.6113826388183,70.)) ;
#43716=CARTESIAN_POINT('',(-3.67300342852949,32.5988070586048,70.)) ;
#43717=CARTESIAN_POINT('',(-5.10980147083728E-14,28.9873448468396,70.)) ;
#43718=CARTESIAN_POINT('Origin',(-2.39808173319034E-14,31.,70.)) ;
#43719=CARTESIAN_POINT('Origin',(-2.39808173319034E-14,31.,70.)) ;
#43720=CARTESIAN_POINT('Origin',(3.44907447632287,30.6113826388183,70.)) ;
#43721=CARTESIAN_POINT('',(6.45029104823248,28.2605715912239,70.)) ;
#43722=CARTESIAN_POINT('',(3.22514552411626,28.6239582190318,70.)) ;
#43723=CARTESIAN_POINT('Origin',(6.89814895264572,30.2227652776365,70.)) ;
#43724=CARTESIAN_POINT('Origin',(6.89814895264572,30.2227652776365,70.)) ;
#43725=CARTESIAN_POINT('Origin',(10.174272432645,29.0764000913058,70.)) ;
#43726=CARTESIAN_POINT('',(12.5771375692369,26.1166952701541,70.)) ;
#43727=CARTESIAN_POINT('',(9.51371430873469,27.188633430689,70.)) ;
#43728=CARTESIAN_POINT('Origin',(13.4503959126443,27.930034904975,70.)) ;
#43729=CARTESIAN_POINT('Origin',(13.4503959126443,27.930034904975,70.)) ;
#43730=CARTESIAN_POINT('Origin',(16.3892898851325,26.083405430742,70.)) ;
#43731=CARTESIAN_POINT('',(18.0733138949668,22.6632187944167,70.)) ;
#43732=CARTESIAN_POINT('',(15.3252257321019,24.3899570322854,70.)) ;
#43733=CARTESIAN_POINT('Origin',(19.3281838576207,24.2367759565089,70.)) ;
#43734=CARTESIAN_POINT('Origin',(19.3281838576207,24.2367759565089,70.)) ;
#43735=CARTESIAN_POINT('Origin',(21.7824799070648,21.7824799070648,70.)) ;
#43736=CARTESIAN_POINT('',(22.6632187944166,18.0733138949668,70.)) ;
#43737=CARTESIAN_POINT('',(20.3682663446917,20.3682663446917,70.)) ;
#43738=CARTESIAN_POINT('Origin',(24.2367759565089,19.3281838576207,70.)) ;
#43739=CARTESIAN_POINT('Origin',(24.2367759565089,19.3281838576207,70.)) ;
#43740=CARTESIAN_POINT('Origin',(26.083405430742,16.3892898851325,70.)) ;
#43741=CARTESIAN_POINT('',(26.1166952701541,12.5771375692369,70.)) ;
#43742=CARTESIAN_POINT('',(24.3899570322854,15.3252257321018,70.)) ;
#43743=CARTESIAN_POINT('Origin',(27.930034904975,13.4503959126443,70.)) ;
#43744=CARTESIAN_POINT('Origin',(27.930034904975,13.4503959126443,70.)) ;
#43745=CARTESIAN_POINT('Origin',(29.0764000913058,10.174272432645,70.)) ;
#43746=CARTESIAN_POINT('',(28.2605715912239,6.45029104823255,70.)) ;
#43747=CARTESIAN_POINT('',(27.188633430689,9.51371430873469,70.)) ;
#43748=CARTESIAN_POINT('Origin',(30.2227652776365,6.89814895264576,70.)) ;
#43749=CARTESIAN_POINT('Origin',(30.2227652776365,6.89814895264576,70.)) ;
#43750=CARTESIAN_POINT('Origin',(30.6113826388183,3.44907447632287,70.)) ;
#43751=CARTESIAN_POINT('',(28.6239582190318,3.22514552411626,70.)) ;
#50341=UNCERTAINTY_MEASURE_WITH_UNIT(LENGTH_MEASURE(0.001),#50441,
'DISTANCE_ACCURACY_VALUE',
'Maximum model space distance between geometric entities at asserted c
onnectivities') ;
#50387=UNCERTAINTY_MEASURE_WITH_UNIT(LENGTH_MEASURE(0.001),#50441,
'DISTANCE_ACCURACY_VALUE',
'Maximum model space distance between geometric entities at asserted c
onnectivities') ;
#50394=(
GEOMETRIC_REPRESENTATION_CONTEXT(3)
GLOBAL_UNCERTAINTY_ASSIGNED_CONTEXT((#50341))
GLOBAL_UNIT_ASSIGNED_CONTEXT((#50441,#50443,#50444))
REPRESENTATION_CONTEXT('','3D')
) ;
#50440=(
GEOMETRIC_REPRESENTATION_CONTEXT(3)
GLOBAL_UNCERTAINTY_ASSIGNED_CONTEXT((#50387))
GLOBAL_UNIT_ASSIGNED_CONTEXT((#50441,#50443,#50444))
REPRESENTATION_CONTEXT('','3D')
) ;
#50441=(
LENGTH_UNIT()
NAMED_UNIT(*)
SI_UNIT(.CENTI.,.METRE.)
) ;
#50443=(
NAMED_UNIT(*)
PLANE_ANGLE_UNIT()
SI_UNIT($,.RADIAN.)
) ;
#50444=(
NAMED_UNIT(*)
SI_UNIT($,.STERADIAN.)
SOLID_ANGLE_UNIT()
) ;
#50451=SHAPE_DEFINITION_REPRESENTATION(#50503,#50625) ;
#50503=PRODUCT_DEFINITION_SHAPE('',$,#50678) ;
#50625=SHAPE_REPRESENTATION('',(#29730),#50394) ;
#50671=PRODUCT_DEFINITION_CONTEXT('part definition',#50829,'design') ;
#50678=PRODUCT_DEFINITION('HOPPER_SUPPORT_RING',
'HOPPER_SUPPORT_RING',#50730,#50671) ;
#50730=PRODUCT_DEFINITION_FORMATION('',$,#50837) ;
#50829=APPLICATION_CONTEXT(
'Core Data for Automotive Mechanical Design Process') ;
#50830=PRODUCT_CONTEXT('part definition',#50829,'mechanical') ;
#50837=PRODUCT('HOPPER_SUPPORT_RING','HOPPER_SUPPORT_RING',$,(#50830)) ;
#50883=PRESENTATION_STYLE_ASSIGNMENT((#50890)) ;
#50890=SURFACE_STYLE_USAGE(.BOTH.,#50897) ;
#50897=SURFACE_SIDE_STYLE('',(#50904)) ;
#50904=SURFACE_STYLE_FILL_AREA(#50911) ;
#50911=FILL_AREA_STYLE('Steel - Satin',(#50918)) ;
#50918=FILL_AREA_STYLE_COLOUR('Steel - Satin',#50925) ;
#50925=COLOUR_RGB('Steel - Satin', 0.31764706, 0.68627451, 0.89019608) ;
ENDSEC;
END-ISO-10303-21;
